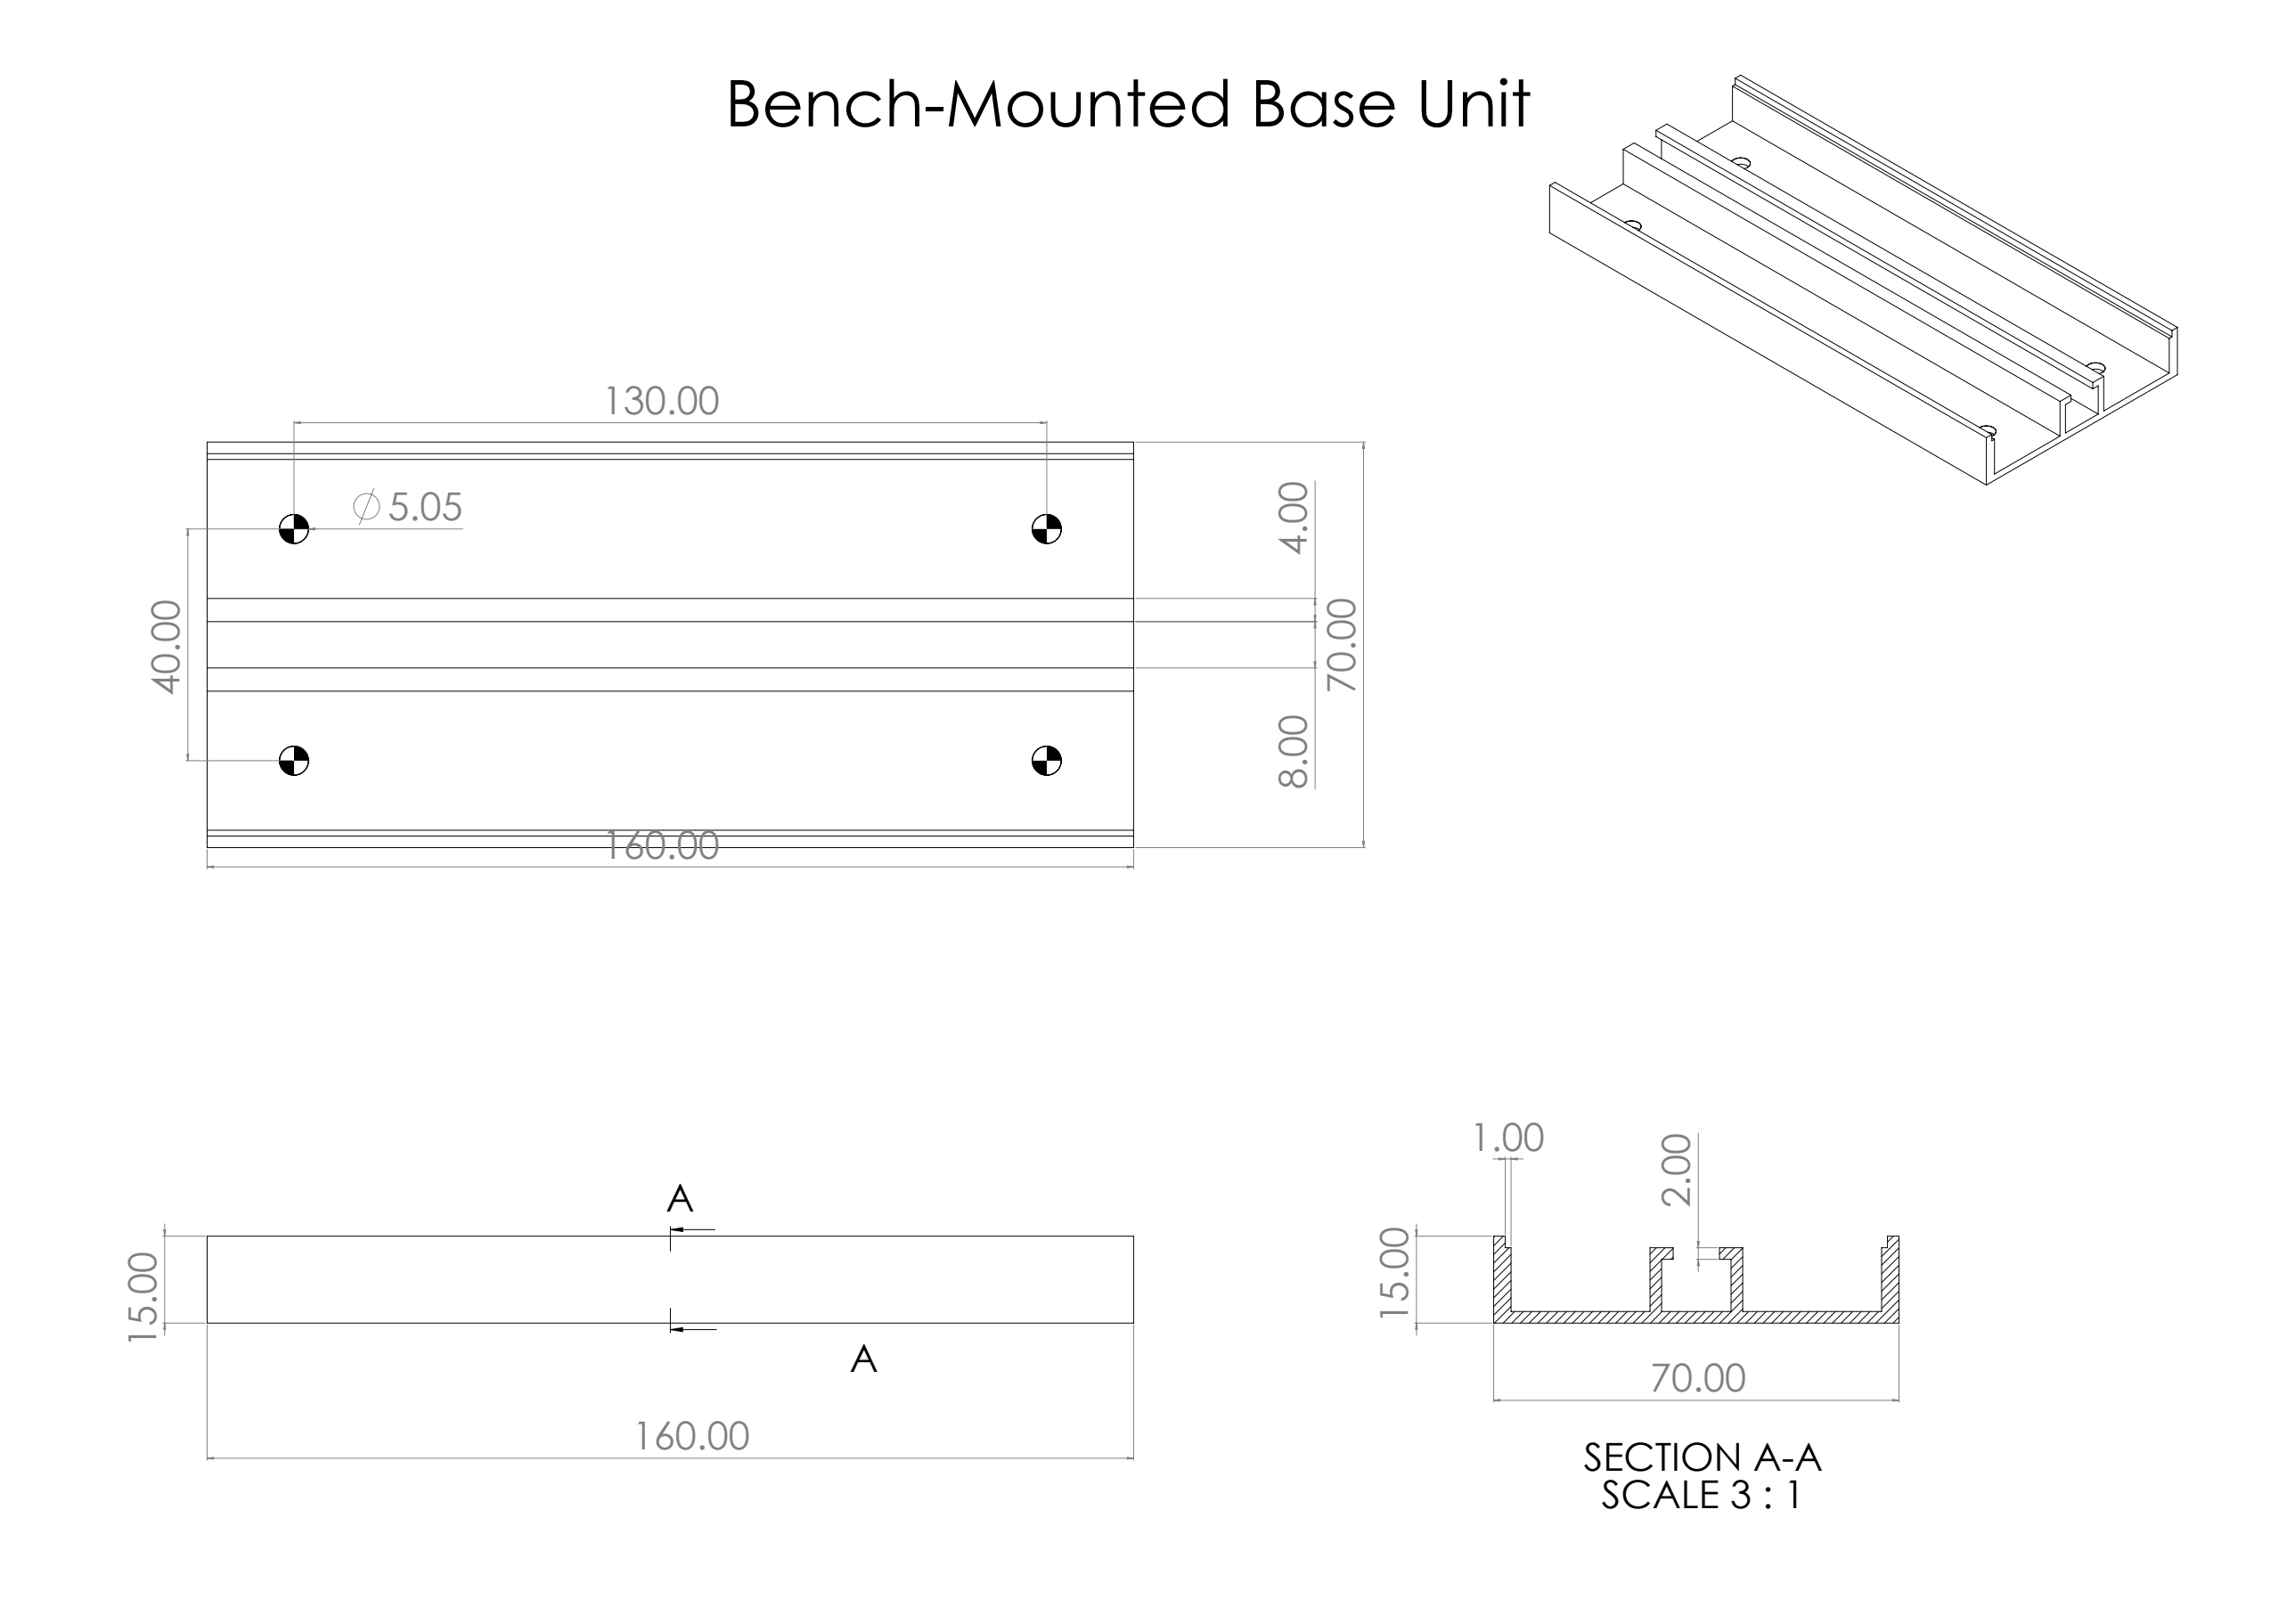
ISO-10303-21;
HEADER;
FILE_DESCRIPTION (('STEP AP214'),
    '1' );
FILE_NAME ('Bench-Mounted Base Unit.step',
    '2026-10-24T21:31:31',
    ( '' ),
    ( '' ),
    'SwSTEP 2.0',
    'SolidWorks 2025',
    '' );
FILE_SCHEMA (( 'AUTOMOTIVE_DESIGN' ));
ENDSEC;

DATA;
#19=ADVANCED_FACE ( 'NONE', ( #7663 ), #4110, .F. ) ;
#25=LINE ( 'NONE', #2406, #7510 ) ;
#36=DIRECTION ( 'NONE',  ( 0.000000000000000000, 0.000000000000000000, 1.000000000000000000 ) ) ;
#50=LINE ( 'NONE', #1350, #13702 ) ;
#81=VERTEX_POINT ( 'NONE', #9278 ) ;
#87=LINE ( 'NONE', #2465, #13317 ) ;
#98=ORIENTED_EDGE ( 'NONE', *, *, #8570, .T. ) ;
#157=EDGE_CURVE ( 'NONE', #531, #1580, #7972, .T. ) ;
#158=ADVANCED_FACE ( 'NONE', ( #10353 ), #436, .F. ) ;
#167=DIRECTION ( 'NONE',  ( -1.000000000000000000, 0.000000000000000000, 0.000000000000000000 ) ) ;
#177=AXIS2_PLACEMENT_3D ( 'NONE', #1271, #10901, #2354 ) ;
#186=EDGE_LOOP ( 'NONE', ( #1865, #4805, #14383, #1234 ) ) ;
#189=PRODUCT_DEFINITION_FORMATION_WITH_SPECIFIED_SOURCE ( 'ANY', '', #5935, .NOT_KNOWN. ) ;
#190=DIRECTION ( 'NONE',  ( -1.000000000000000000, -0.000000000000000000, -0.000000000000000000 ) ) ;
#205=ADVANCED_FACE ( 'NONE', ( #8045 ), #8050, .F. ) ;
#206=AXIS2_PLACEMENT_3D ( 'NONE', #6103, #12884, #8338 ) ;
#224=ORIENTED_EDGE ( 'NONE', *, *, #5040, .T. ) ;
#227=ORIENTED_EDGE ( 'NONE', *, *, #14224, .F. ) ;
#237=ORIENTED_EDGE ( 'NONE', *, *, #6908, .T. ) ;
#246=VERTEX_POINT ( 'NONE', #9730 ) ;
#280=LINE ( 'NONE', #11038, #4450 ) ;
#288=DIRECTION ( 'NONE',  ( 0.000000000000000000, -0.000000000000000000, -1.000000000000000000 ) ) ;
#292=EDGE_CURVE ( 'NONE', #5596, #3737, #9002, .T. ) ;
#295=ADVANCED_FACE ( 'NONE', ( #10164 ), #9788, .F. ) ;
#307=VERTEX_POINT ( 'NONE', #9085 ) ;
#313=CARTESIAN_POINT ( 'NONE',  ( 65.00000000000001421, -85.24929059928631148, 19.99999999999999645 ) ) ;
#341=VERTEX_POINT ( 'NONE', #685 ) ;
#395=EDGE_CURVE ( 'NONE', #2944, #14405, #10471, .T. ) ;
#404=VERTEX_POINT ( 'NONE', #7006 ) ;
#436=CONICAL_SURFACE ( 'NONE', #4856, 2.524999999999999467, 0.7853981633973787790 ) ;
#446=VERTEX_POINT ( 'NONE', #13931 ) ;
#450=EDGE_LOOP ( 'NONE', ( #14518, #14522, #9749, #6218 ) ) ;
#466=ADVANCED_FACE ( 'NONE', ( #3619 ), #3388, .F. ) ;
#475=VECTOR ( 'NONE', #11454, 1000.000000000000000 ) ;
#494=CARTESIAN_POINT ( 'NONE',  ( 80.00000000000001421, -72.24929059928631148, -32.99999999999999289 ) ) ;
#504=DIRECTION ( 'NONE',  ( -0.000000000000000000, 1.000000000000000000, 1.445602896647339163E-16 ) ) ;
#507=CARTESIAN_POINT ( 'NONE',  ( -80.00000000000001421, -74.24929059928631148, 8.000000000000001776 ) ) ;
#519=CARTESIAN_POINT ( 'NONE',  ( -80.00000000000001421, -72.24929059928631148, -32.99999999999999289 ) ) ;
#521=ORIENTED_EDGE ( 'NONE', *, *, #7499, .F. ) ;
#523=FACE_OUTER_BOUND ( 'NONE', #7005, .T. ) ;
#531=VERTEX_POINT ( 'NONE', #1686 ) ;
#538=VERTEX_POINT ( 'NONE', #9636 ) ;
#566=AXIS2_PLACEMENT_3D ( 'NONE', #4908, #5202, #14225 ) ;
#570=EDGE_CURVE ( 'NONE', #1671, #7867, #6379, .T. ) ;
#586=ORIENTED_EDGE ( 'NONE', *, *, #12573, .F. ) ;
#590=DIRECTION ( 'NONE',  ( 0.000000000000000000, 0.000000000000000000, 1.000000000000000000 ) ) ;
#592=DIRECTION ( 'NONE',  ( 0.000000000000000000, 0.7071067811865965336, 0.7071067811864985009 ) ) ;
#595=ADVANCED_FACE ( 'NONE', ( #523 ), #13090, .F. ) ;
#605=ORIENTED_EDGE ( 'NONE', *, *, #6309, .T. ) ;
#606=DIRECTION ( 'NONE',  ( -0.000000000000000000, 1.000000000000000000, 1.445602896647339163E-16 ) ) ;
#608=PLANE ( 'NONE',  #3506 ) ;
#634=DIRECTION ( 'NONE',  ( 0.000000000000000000, -0.000000000000000000, 1.000000000000000000 ) ) ;
#638=FACE_OUTER_BOUND ( 'NONE', #15061, .T. ) ;
#645=EDGE_CURVE ( 'NONE', #11420, #3697, #6168, .T. ) ;
#649=DIRECTION ( 'NONE',  ( 0.000000000000000000, 0.000000000000000000, -1.000000000000000000 ) ) ;
#671=CIRCLE ( 'NONE', #2885, 2.524999999999999467 ) ;
#685=CARTESIAN_POINT ( 'NONE',  ( -80.00000000000001421, -85.24929059928631148, 6.000000000000001776 ) ) ;
#699=ORIENTED_EDGE ( 'NONE', *, *, #13284, .T. ) ;
#712=DIRECTION ( 'NONE',  ( 8.659560562354330119E-17, 0.7071067811865966446, -0.7071067811864982788 ) ) ;
#715=EDGE_LOOP ( 'NONE', ( #1135, #7087, #13779, #14842 ) ) ;
#717=ORIENTED_EDGE ( 'NONE', *, *, #12868, .T. ) ;
#723=DIRECTION ( 'NONE',  ( 0.000000000000000000, 0.000000000000000000, 1.000000000000000000 ) ) ;
#725=AXIS2_PLACEMENT_3D ( 'NONE', #10060, #14667, #13517 ) ;
#726=ORIENTED_EDGE ( 'NONE', *, *, #9673, .T. ) ;
#732=CARTESIAN_POINT ( 'NONE',  ( 80.00000000000001421, -85.24929059928629727, -8.000000000000001776 ) ) ;
#733=DIRECTION ( 'NONE',  ( -1.000000000000000000, -0.000000000000000000, -0.000000000000000000 ) ) ;
#737=EDGE_CURVE ( 'NONE', #9321, #13009, #5442, .T. ) ;
#747=ORIENTED_EDGE ( 'NONE', *, *, #4471, .F. ) ;
#777=VERTEX_POINT ( 'NONE', #2331 ) ;
#784=VECTOR ( 'NONE', #14829, 1000.000000000000000 ) ;
#793=DIRECTION ( 'NONE',  ( -0.000000000000000000, 1.000000000000000000, 1.445602896647339163E-16 ) ) ;
#824=DIRECTION ( 'NONE',  ( 1.000000000000000000, 0.000000000000000000, 0.000000000000000000 ) ) ;
#831=ORIENTED_EDGE ( 'NONE', *, *, #11996, .T. ) ;
#839=DIRECTION ( 'NONE',  ( -0.000000000000000000, 0.000000000000000000, 1.000000000000000000 ) ) ;
#841=ADVANCED_FACE ( 'NONE', ( #12100 ), #14411, .F. ) ;
#866=VECTOR ( 'NONE', #2481, 1000.000000000000000 ) ;
#893=CARTESIAN_POINT ( 'NONE',  ( 65.00000000000001421, -87.24929059928631148, -19.99999999999999645 ) ) ;
#917=CARTESIAN_POINT ( 'NONE',  ( 65.00000000000001421, -85.24929059928629727, -19.99999999999999645 ) ) ;
#935=CARTESIAN_POINT ( 'NONE',  ( 80.00000000000001421, -74.24929059928631148, -4.000000000000000000 ) ) ;
#938=CARTESIAN_POINT ( 'NONE',  ( -65.00000000000001421, -85.24929059928629727, -19.99999999999999645 ) ) ;
#950=EDGE_CURVE ( 'NONE', #9272, #7803, #4209, .T. ) ;
#951=LINE ( 'NONE', #6885, #9647 ) ;
#960=CYLINDRICAL_SURFACE ( 'NONE', #11471, 2.499999999999995115 ) ;
#979=ORIENTED_EDGE ( 'NONE', *, *, #14140, .T. ) ;
#989=ADVANCED_FACE ( 'NONE', ( #7762 ), #6601, .F. ) ;
#995=DIRECTION ( 'NONE',  ( -1.000000000000000000, -0.000000000000000000, -0.000000000000000000 ) ) ;
#1008=FACE_OUTER_BOUND ( 'NONE', #715, .T. ) ;
#1018=LINE ( 'NONE', #2095, #4193 ) ;
#1029=DIRECTION ( 'NONE',  ( 0.000000000000000000, -1.000000000000000000, 1.927470528863120035E-16 ) ) ;
#1038=VECTOR ( 'NONE', #8723, 1000.000000000000000 ) ;
#1042=ORIENTED_EDGE ( 'NONE', *, *, #3581, .T. ) ;
#1046=VECTOR ( 'NONE', #9005, 1000.000000000000000 ) ;
#1058=DIRECTION ( 'NONE',  ( -0.000000000000000000, -1.000000000000000000, 4.625929269271485914E-16 ) ) ;
#1071=PLANE ( 'NONE',  #4829 ) ;
#1083=VERTEX_POINT ( 'NONE', #14148 ) ;
#1090=LINE ( 'NONE', #3173, #14166 ) ;
#1095=CARTESIAN_POINT ( 'NONE',  ( -80.00000000000001421, -74.24929059928631148, 32.99999999999999289 ) ) ;
#1135=ORIENTED_EDGE ( 'NONE', *, *, #12418, .T. ) ;
#1182=DIRECTION ( 'NONE',  ( 0.000000000000000000, 0.000000000000000000, 1.000000000000000000 ) ) ;
#1183=CIRCLE ( 'NONE', #7088, 2.499999999999995115 ) ;
#1184=VERTEX_POINT ( 'NONE', #1443 ) ;
#1186=EDGE_LOOP ( 'NONE', ( #7240, #3544 ) ) ;
#1209=LINE ( 'NONE', #4592, #1781 ) ;
#1234=ORIENTED_EDGE ( 'NONE', *, *, #15073, .T. ) ;
#1237=EDGE_CURVE ( 'NONE', #11933, #12860, #5235, .T. ) ;
#1245=ORIENTED_EDGE ( 'NONE', *, *, #645, .F. ) ;
#1246=DIRECTION ( 'NONE',  ( 0.000000000000000000, 0.000000000000000000, 1.000000000000000000 ) ) ;
#1271=CARTESIAN_POINT ( 'NONE',  ( 80.00000000000001421, -85.24929059928629727, 32.00000000000000000 ) ) ;
#1274=ORIENTED_EDGE ( 'NONE', *, *, #4240, .F. ) ;
#1285=VECTOR ( 'NONE', #3850, 1000.000000000000000 ) ;
#1296=EDGE_CURVE ( 'NONE', #3181, #6626, #5246, .T. ) ;
#1311=VERTEX_POINT ( 'NONE', #9697 ) ;
#1316=FACE_OUTER_BOUND ( 'NONE', #2115, .T. ) ;
#1323=ORIENTED_EDGE ( 'NONE', *, *, #13700, .F. ) ;
#1329=ADVANCED_FACE ( 'NONE', ( #5059 ), #3895, .F. ) ;
#1330=DIRECTION ( 'NONE',  ( -1.000000000000000000, -0.000000000000000000, -0.000000000000000000 ) ) ;
#1350=CARTESIAN_POINT ( 'NONE',  ( 80.00000000000001421, -85.24929059928629727, 8.000000000000001776 ) ) ;
#1389=ORIENTED_EDGE ( 'NONE', *, *, #12424, .F. ) ;
#1407=ADVANCED_FACE ( 'NONE', ( #7894 ), #8810, .F. ) ;
#1413=CARTESIAN_POINT ( 'NONE',  ( 80.00000000000001421, -76.24929059928631148, -6.000000000000000000 ) ) ;
#1417=FACE_OUTER_BOUND ( 'NONE', #2786, .T. ) ;
#1430=EDGE_CURVE ( 'NONE', #4665, #307, #15084, .T. ) ;
#1443=CARTESIAN_POINT ( 'NONE',  ( -80.00000000000001421, -76.24929059928631148, -6.000000000000000000 ) ) ;
#1452=AXIS2_PLACEMENT_3D ( 'NONE', #11065, #9559, #2549 ) ;
#1456=ORIENTED_EDGE ( 'NONE', *, *, #10701, .T. ) ;
#1465=DIRECTION ( 'NONE',  ( 0.000000000000000000, -1.000000000000000000, 0.000000000000000000 ) ) ;
#1466=DIRECTION ( 'NONE',  ( -1.000000000000000000, -0.000000000000000000, -0.000000000000000000 ) ) ;
#1471=VECTOR ( 'NONE', #995, 1000.000000000000000 ) ;
#1479=EDGE_CURVE ( 'NONE', #5596, #6896, #5906, .T. ) ;
#1480=DIRECTION ( 'NONE',  ( -0.000000000000000000, 1.000000000000000000, 1.445602896647339163E-16 ) ) ;
#1490=DIRECTION ( 'NONE',  ( -0.000000000000000000, 1.000000000000000000, -0.000000000000000000 ) ) ;
#1491=CARTESIAN_POINT ( 'NONE',  ( 65.00000000000001421, -85.24929059928629727, -22.52499999999999503 ) ) ;
#1552=CARTESIAN_POINT ( 'NONE',  ( 80.00000000000001421, -76.24929059928631148, -4.000000000000000000 ) ) ;
#1571=( NAMED_UNIT ( * ) PLANE_ANGLE_UNIT ( ) SI_UNIT ( $, .RADIAN. ) );
#1580=VERTEX_POINT ( 'NONE', #13813 ) ;
#1584=DIRECTION ( 'NONE',  ( -1.000000000000000000, -0.000000000000000000, -0.000000000000000000 ) ) ;
#1589=PLANE ( 'NONE',  #10650 ) ;
#1604=EDGE_CURVE ( 'NONE', #12366, #3697, #9209, .T. ) ;
#1615=ORIENTED_EDGE ( 'NONE', *, *, #2520, .F. ) ;
#1636=( NAMED_UNIT ( * ) SI_UNIT ( $, .STERADIAN. ) SOLID_ANGLE_UNIT ( ) );
#1638=SHAPE_REPRESENTATION_RELATIONSHIP ( 'NONE' , 'NONE' ,  #11466, #10707 ) ;
#1644=AXIS2_PLACEMENT_3D ( 'NONE', #14275, #15068, #3574 ) ;
#1645=AXIS2_PLACEMENT_3D ( 'NONE', #14043, #15199, #1029 ) ;
#1668=VECTOR ( 'NONE', #10391, 1000.000000000000000 ) ;
#1671=VERTEX_POINT ( 'NONE', #11398 ) ;
#1683=ORIENTED_EDGE ( 'NONE', *, *, #7122, .F. ) ;
#1686=CARTESIAN_POINT ( 'NONE',  ( -80.00000000000001421, -74.24929059928631148, -8.000000000000001776 ) ) ;
#1689=EDGE_LOOP ( 'NONE', ( #1895, #13919 ) ) ;
#1696=DIRECTION ( 'NONE',  ( 0.000000000000000000, 1.000000000000000000, 0.000000000000000000 ) ) ;
#1706=VECTOR ( 'NONE', #9108, 1000.000000000000000 ) ;
#1722=ORIENTED_EDGE ( 'NONE', *, *, #13799, .T. ) ;
#1724=CARTESIAN_POINT ( 'NONE',  ( 80.00000000000001421, -85.24929059928631148, -6.000000000000001776 ) ) ;
#1745=AXIS2_PLACEMENT_3D ( 'NONE', #3312, #839, #5548 ) ;
#1750=CARTESIAN_POINT ( 'NONE',  ( 65.00000000000001421, -87.24929059928631148, -17.50000000000000000 ) ) ;
#1752=ORIENTED_EDGE ( 'NONE', *, *, #14178, .F. ) ;
#1758=ORIENTED_EDGE ( 'NONE', *, *, #7122, .T. ) ;
#1766=VECTOR ( 'NONE', #7495, 1000.000000000000000 ) ;
#1781=VECTOR ( 'NONE', #5838, 1000.000000000000000 ) ;
#1800=VECTOR ( 'NONE', #3512, 1000.000000000000000 ) ;
#1814=CARTESIAN_POINT ( 'NONE',  ( 80.00000000000001421, -74.24929059928631148, 32.00000000000000000 ) ) ;
#1825=DIRECTION ( 'NONE',  ( -1.000000000000000000, -0.000000000000000000, -0.000000000000000000 ) ) ;
#1827=LINE ( 'NONE', #519, #6922 ) ;
#1843=EDGE_CURVE ( 'NONE', #3737, #2170, #10798, .T. ) ;
#1859=DIRECTION ( 'NONE',  ( -1.000000000000000000, -0.000000000000000000, -0.000000000000000000 ) ) ;
#1863=VERTEX_POINT ( 'NONE', #9494 ) ;
#1865=ORIENTED_EDGE ( 'NONE', *, *, #645, .T. ) ;
#1878=VECTOR ( 'NONE', #4733, 1000.000000000000000 ) ;
#1880=FACE_OUTER_BOUND ( 'NONE', #12072, .T. ) ;
#1888=EDGE_LOOP ( 'NONE', ( #8253, #2831, #13213, #11548 ) ) ;
#1895=ORIENTED_EDGE ( 'NONE', *, *, #14224, .T. ) ;
#1917=CARTESIAN_POINT ( 'NONE',  ( 80.00000000000001421, -85.24929059928629727, -32.00000000000000000 ) ) ;
#1918=VERTEX_POINT ( 'NONE', #4502 ) ;
#1919=DIRECTION ( 'NONE',  ( 0.000000000000000000, 0.000000000000000000, 1.000000000000000000 ) ) ;
#1937=VECTOR ( 'NONE', #1859, 1000.000000000000000 ) ;
#1966=CARTESIAN_POINT ( 'NONE',  ( 80.00000000000001421, -74.24929059928631148, 4.000000000000000000 ) ) ;
#1978=VERTEX_POINT ( 'NONE', #9357 ) ;
#1999=VECTOR ( 'NONE', #1490, 1000.000000000000000 ) ;
#2012=AXIS2_PLACEMENT_3D ( 'NONE', #10249, #6482, #7789 ) ;
#2026=VECTOR ( 'NONE', #8584, 1000.000000000000000 ) ;
#2032=LINE ( 'NONE', #10277, #9994 ) ;
#2049=CARTESIAN_POINT ( 'NONE',  ( -65.00000000000001421, -85.24929059928631148, 19.99999999999999645 ) ) ;
#2050=ORIENTED_EDGE ( 'NONE', *, *, #12034, .T. ) ;
#2054=DIRECTION ( 'NONE',  ( -1.000000000000000000, -0.000000000000000000, -0.000000000000000000 ) ) ;
#2060=DIRECTION ( 'NONE',  ( 8.659560562354330119E-17, 0.7071067811865966446, -0.7071067811864982788 ) ) ;
#2095=CARTESIAN_POINT ( 'NONE',  ( 80.00000000000001421, -74.24929059928631148, -8.000000000000001776 ) ) ;
#2110=CARTESIAN_POINT ( 'NONE',  ( -65.00000000000001421, -85.24929059928631148, 19.99999999999999645 ) ) ;
#2115=EDGE_LOOP ( 'NONE', ( #2607, #14282, #14380, #13821 ) ) ;
#2126=CARTESIAN_POINT ( 'NONE',  ( -80.00000000000001421, -74.24929059928631148, -32.99999999999999289 ) ) ;
#2127=CARTESIAN_POINT ( 'NONE',  ( 80.00000000000001421, -74.24929059928631148, 32.99999999999999289 ) ) ;
#2142=CARTESIAN_POINT ( 'NONE',  ( 65.00000000000001421, -87.24929059928631148, -19.99999999999999645 ) ) ;
#2151=DIRECTION ( 'NONE',  ( 0.000000000000000000, 1.000000000000000000, 1.927470528863120035E-16 ) ) ;
#2153=CARTESIAN_POINT ( 'NONE',  ( 80.00000000000001421, -85.24929059928629727, 32.00000000000000000 ) ) ;
#2158=ORIENTED_EDGE ( 'NONE', *, *, #4168, .T. ) ;
#2164=DIRECTION ( 'NONE',  ( -0.000000000000000000, 1.000000000000000000, 1.445602896647339163E-16 ) ) ;
#2170=VERTEX_POINT ( 'NONE', #14207 ) ;
#2186=CARTESIAN_POINT ( 'NONE',  ( 65.00000000000001421, -85.27429059928630295, 22.50000000000000000 ) ) ;
#2202=CARTESIAN_POINT ( 'NONE',  ( -80.00000000000001421, -72.24929059928631148, 34.99999999999999289 ) ) ;
#2222=DIRECTION ( 'NONE',  ( 0.000000000000000000, 1.000000000000000000, 0.000000000000000000 ) ) ;
#2246=DIRECTION ( 'NONE',  ( 0.000000000000000000, -1.000000000000000000, -4.625929269271485914E-16 ) ) ;
#2249=DIRECTION ( 'NONE',  ( 0.000000000000000000, 0.000000000000000000, 1.000000000000000000 ) ) ;
#2268=CIRCLE ( 'NONE', #10878, 2.524999999999999467 ) ;
#2279=ADVANCED_FACE ( 'NONE', ( #7007 ), #14950, .F. ) ;
#2290=CARTESIAN_POINT ( 'NONE',  ( -65.00000000000001421, -85.24929059928629727, -19.99999999999999645 ) ) ;
#2293=VECTOR ( 'NONE', #12378, 1000.000000000000114 ) ;
#2310=ADVANCED_FACE ( 'NONE', ( #5628 ), #10397, .F. ) ;
#2322=DIRECTION ( 'NONE',  ( 0.000000000000000000, 0.000000000000000000, 1.000000000000000000 ) ) ;
#2330=CARTESIAN_POINT ( 'NONE',  ( 65.00000000000001421, -85.24929059928631148, 17.50000000000000000 ) ) ;
#2331=CARTESIAN_POINT ( 'NONE',  ( -65.00000000000001421, -85.24929059928631148, 22.52499999999999503 ) ) ;
#2344=LINE ( 'NONE', #3502, #12602 ) ;
#2354=DIRECTION ( 'NONE',  ( 0.000000000000000000, -1.445602896647339410E-16, -1.000000000000000000 ) ) ;
#2355=ADVANCED_FACE ( 'NONE', ( #12549 ), #6693, .F. ) ;
#2357=EDGE_CURVE ( 'NONE', #2753, #3972, #8006, .T. ) ;
#2380=CARTESIAN_POINT ( 'NONE',  ( 80.00000000000001421, -76.24929059928631148, 4.000000000000000000 ) ) ;
#2382=EDGE_LOOP ( 'NONE', ( #1456, #9704, #14086, #14524 ) ) ;
#2406=CARTESIAN_POINT ( 'NONE',  ( 80.00000000000001421, -76.24929059928631148, -6.000000000000000000 ) ) ;
#2419=DIRECTION ( 'NONE',  ( -0.000000000000000000, 1.000000000000000000, 1.445602896647339163E-16 ) ) ;
#2465=CARTESIAN_POINT ( 'NONE',  ( -80.00000000000001421, -85.24929059928629727, -32.00000000000000000 ) ) ;
#2471=CARTESIAN_POINT ( 'NONE',  ( 80.00000000000001421, -76.24929059928631148, 4.000000000000000000 ) ) ;
#2481=DIRECTION ( 'NONE',  ( -0.000000000000000000, -0.000000000000000000, 1.000000000000000000 ) ) ;
#2487=AXIS2_PLACEMENT_3D ( 'NONE', #5138, #3973, #3903 ) ;
#2491=ORIENTED_EDGE ( 'NONE', *, *, #11907, .T. ) ;
#2520=EDGE_CURVE ( 'NONE', #10741, #11420, #9637, .T. ) ;
#2525=VECTOR ( 'NONE', #2575, 1000.000000000000000 ) ;
#2547=EDGE_LOOP ( 'NONE', ( #6515, #3993 ) ) ;
#2549=DIRECTION ( 'NONE',  ( 0.000000000000000000, 1.000000000000000000, -4.625929269271485914E-16 ) ) ;
#2567=FACE_OUTER_BOUND ( 'NONE', #7297, .T. ) ;
#2575=DIRECTION ( 'NONE',  ( 0.000000000000000000, 0.000000000000000000, -1.000000000000000000 ) ) ;
#2577=CARTESIAN_POINT ( 'NONE',  ( -65.00000000000001421, -85.24929059928631148, 17.50000000000000000 ) ) ;
#2586=UNCERTAINTY_MEASURE_WITH_UNIT (LENGTH_MEASURE( 1.000000000000000082E-05 ), #3939, 'distance_accuracy_value', 'NONE');
#2589=VERTEX_POINT ( 'NONE', #12224 ) ;
#2601=EDGE_CURVE ( 'NONE', #14307, #7867, #11002, .T. ) ;
#2607=ORIENTED_EDGE ( 'NONE', *, *, #6790, .F. ) ;
#2670=EDGE_LOOP ( 'NONE', ( #15221, #586, #6959, #4327 ) ) ;
#2675=ORIENTED_EDGE ( 'NONE', *, *, #5963, .T. ) ;
#2677=CARTESIAN_POINT ( 'NONE',  ( -65.00000000000001421, -85.24929059928631148, 17.47499999999999787 ) ) ;
#2679=PLANE ( 'NONE',  #2487 ) ;
#2698=ORIENTED_EDGE ( 'NONE', *, *, #14591, .F. ) ;
#2700=LINE ( 'NONE', #1552, #4226 ) ;
#2720=DIRECTION ( 'NONE',  ( 0.000000000000000000, -0.000000000000000000, -1.000000000000000000 ) ) ;
#2729=UNCERTAINTY_MEASURE_WITH_UNIT (LENGTH_MEASURE( 1.000000000000000082E-05 ), #6118, 'distance_accuracy_value', 'NONE');
#2731=DIRECTION ( 'NONE',  ( -0.000000000000000000, 1.000000000000000000, 1.445602896647339163E-16 ) ) ;
#2751=ORIENTED_EDGE ( 'NONE', *, *, #10179, .F. ) ;
#2753=VERTEX_POINT ( 'NONE', #5431 ) ;
#2781=CARTESIAN_POINT ( 'NONE',  ( -80.00000000000001421, -87.24929059928629727, 0.000000000000000000 ) ) ;
#2786=EDGE_LOOP ( 'NONE', ( #13073, #9483, #7592, #3260 ) ) ;
#2804=CARTESIAN_POINT ( 'NONE',  ( 80.00000000000001421, -76.24929059928631148, 6.000000000000000000 ) ) ;
#2831=ORIENTED_EDGE ( 'NONE', *, *, #1296, .F. ) ;
#2845=FACE_OUTER_BOUND ( 'NONE', #7939, .T. ) ;
#2885=AXIS2_PLACEMENT_3D ( 'NONE', #3967, #504, #14517 ) ;
#2892=DIRECTION ( 'NONE',  ( 1.000000000000000000, 0.000000000000000000, 0.000000000000000000 ) ) ;
#2923=EDGE_CURVE ( 'NONE', #3601, #1918, #7158, .T. ) ;
#2938=ORIENTED_EDGE ( 'NONE', *, *, #12012, .T. ) ;
#2941=VECTOR ( 'NONE', #5173, 1000.000000000000000 ) ;
#2944=VERTEX_POINT ( 'NONE', #13276 ) ;
#2954=LINE ( 'NONE', #8714, #5680 ) ;
#2965=CARTESIAN_POINT ( 'NONE',  ( 80.00000000000001421, -72.24929059928631148, -34.99999999999999289 ) ) ;
#3011=VERTEX_POINT ( 'NONE', #8791 ) ;
#3018=ORIENTED_EDGE ( 'NONE', *, *, #2923, .F. ) ;
#3022=EDGE_CURVE ( 'NONE', #7867, #1978, #2954, .T. ) ;
#3037=AXIS2_PLACEMENT_3D ( 'NONE', #4264, #11343, #6733 ) ;
#3042=CARTESIAN_POINT ( 'NONE',  ( 80.00000000000001421, -85.24929059928629727, 8.000000000000001776 ) ) ;
#3051=DIRECTION ( 'NONE',  ( 0.000000000000000000, 0.000000000000000000, 1.000000000000000000 ) ) ;
#3066=DIRECTION ( 'NONE',  ( -1.000000000000000000, -0.000000000000000000, -0.000000000000000000 ) ) ;
#3068=EDGE_CURVE ( 'NONE', #3756, #446, #14953, .T. ) ;
#3075=ORIENTED_EDGE ( 'NONE', *, *, #13143, .F. ) ;
#3095=CARTESIAN_POINT ( 'NONE',  ( 80.00000000000001421, -76.24929059928631148, 6.000000000000000000 ) ) ;
#3106=EDGE_CURVE ( 'NONE', #1863, #1580, #7956, .T. ) ;
#3110=VERTEX_POINT ( 'NONE', #3095 ) ;
#3121=ORIENTED_EDGE ( 'NONE', *, *, #3711, .F. ) ;
#3133=VECTOR ( 'NONE', #5474, 1000.000000000000000 ) ;
#3135=CARTESIAN_POINT ( 'NONE',  ( -65.00000000000001421, -85.27429059928630295, 19.99999999999999645 ) ) ;
#3161=CARTESIAN_POINT ( 'NONE',  ( 80.00000000000001421, -72.24929059928631148, 34.99999999999999289 ) ) ;
#3173=CARTESIAN_POINT ( 'NONE',  ( 80.00000000000001421, -74.24929059928631148, 32.00000000000000000 ) ) ;
#3181=VERTEX_POINT ( 'NONE', #11714 ) ;
#3204=CARTESIAN_POINT ( 'NONE',  ( -65.00000000000001421, -85.27429059928630295, 22.50000000000000000 ) ) ;
#3240=ADVANCED_FACE ( 'NONE', ( #2567 ), #10799, .F. ) ;
#3260=ORIENTED_EDGE ( 'NONE', *, *, #14534, .T. ) ;
#3262=VERTEX_POINT ( 'NONE', #12808 ) ;
#3300=DIRECTION ( 'NONE',  ( 0.000000000000000000, 0.000000000000000000, 1.000000000000000000 ) ) ;
#3306=ORIENTED_EDGE ( 'NONE', *, *, #12717, .F. ) ;
#3312=CARTESIAN_POINT ( 'NONE',  ( 80.00000000000001421, -74.24929059928631148, 4.000000000000000000 ) ) ;
#3322=CARTESIAN_POINT ( 'NONE',  ( -80.00000000000001421, -72.24929059928631148, -32.99999999999999289 ) ) ;
#3334=AXIS2_PLACEMENT_3D ( 'NONE', #7174, #8340, #1246 ) ;
#3366=( GEOMETRIC_REPRESENTATION_CONTEXT ( 3 ) GLOBAL_UNCERTAINTY_ASSIGNED_CONTEXT ( ( #2586 ) ) GLOBAL_UNIT_ASSIGNED_CONTEXT ( ( #3939, #1571, #4958 ) ) REPRESENTATION_CONTEXT ( 'NONE', 'WORKASPACE' ) );
#3369=CARTESIAN_POINT ( 'NONE',  ( 80.00000000000001421, -87.24929059928631148, 35.00000000000000000 ) ) ;
#3372=FACE_OUTER_BOUND ( 'NONE', #2382, .T. ) ;
#3385=EDGE_CURVE ( 'NONE', #12875, #1311, #15226, .T. ) ;
#3388=PLANE ( 'NONE',  #14203 ) ;
#3411=DIRECTION ( 'NONE',  ( -1.000000000000000000, 0.000000000000000000, -0.000000000000000000 ) ) ;
#3425=AXIS2_PLACEMENT_3D ( 'NONE', #7024, #3563, #3411 ) ;
#3435=EDGE_CURVE ( 'NONE', #538, #5126, #9087, .T. ) ;
#3502=CARTESIAN_POINT ( 'NONE',  ( 80.00000000000001421, -74.24929059928631148, -32.00000000000000000 ) ) ;
#3506=AXIS2_PLACEMENT_3D ( 'NONE', #8845, #10008, #11079 ) ;
#3512=DIRECTION ( 'NONE',  ( -1.000000000000000000, -0.000000000000000000, -0.000000000000000000 ) ) ;
#3514=DIRECTION ( 'NONE',  ( -0.000000000000000000, -1.000000000000000000, -0.000000000000000000 ) ) ;
#3540=FACE_OUTER_BOUND ( 'NONE', #7300, .T. ) ;
#3544=ORIENTED_EDGE ( 'NONE', *, *, #7499, .T. ) ;
#3563=DIRECTION ( 'NONE',  ( 0.000000000000000000, 0.000000000000000000, -1.000000000000000000 ) ) ;
#3574=DIRECTION ( 'NONE',  ( 0.000000000000000000, -0.000000000000000000, 1.000000000000000000 ) ) ;
#3581=EDGE_CURVE ( 'NONE', #446, #7966, #5251, .T. ) ;
#3589=ORIENTED_EDGE ( 'NONE', *, *, #14866, .F. ) ;
#3599=VECTOR ( 'NONE', #14599, 1000.000000000000000 ) ;
#3600=ORIENTED_EDGE ( 'NONE', *, *, #6884, .T. ) ;
#3601=VERTEX_POINT ( 'NONE', #15015 ) ;
#3602=CONICAL_SURFACE ( 'NONE', #7532, 2.524999999999999467, 0.7853981633973787790 ) ;
#3619=FACE_OUTER_BOUND ( 'NONE', #11346, .T. ) ;
#3622=LINE ( 'NONE', #13311, #11142 ) ;
#3636=CYLINDRICAL_SURFACE ( 'NONE', #206, 2.499999999999995115 ) ;
#3639=LINE ( 'NONE', #2330, #8988 ) ;
#3656=AXIS2_PLACEMENT_3D ( 'NONE', #8168, #9399, #4459 ) ;
#3659=DIRECTION ( 'NONE',  ( 0.000000000000000000, 0.7071067811865965336, 0.7071067811864985009 ) ) ;
#3675=CARTESIAN_POINT ( 'NONE',  ( 65.00000000000001421, -87.24929059928631148, 19.99999999999999645 ) ) ;
#3676=AXIS2_PLACEMENT_3D ( 'NONE', #8702, #5248, #14621 ) ;
#3681=ORIENTED_EDGE ( 'NONE', *, *, #12056, .T. ) ;
#3683=ORIENTED_EDGE ( 'NONE', *, *, #14758, .T. ) ;
#3692=DIRECTION ( 'NONE',  ( -1.000000000000000000, -0.000000000000000000, -0.000000000000000000 ) ) ;
#3697=VERTEX_POINT ( 'NONE', #12766 ) ;
#3699=VECTOR ( 'NONE', #15100, 1000.000000000000000 ) ;
#3711=EDGE_CURVE ( 'NONE', #446, #5596, #11513, .T. ) ;
#3718=DIRECTION ( 'NONE',  ( 0.000000000000000000, -1.000000000000000000, 0.000000000000000000 ) ) ;
#3730=EDGE_CURVE ( 'NONE', #15028, #1311, #13679, .T. ) ;
#3734=AXIS2_PLACEMENT_3D ( 'NONE', #2142, #2222, #3300 ) ;
#3737=VERTEX_POINT ( 'NONE', #12682 ) ;
#3756=VERTEX_POINT ( 'NONE', #12446 ) ;
#3771=DIRECTION ( 'NONE',  ( 0.000000000000000000, 0.000000000000000000, 1.000000000000000000 ) ) ;
#3775=AXIS2_PLACEMENT_3D ( 'NONE', #7091, #5010, #3771 ) ;
#3784=FACE_OUTER_BOUND ( 'NONE', #9288, .T. ) ;
#3794=FACE_OUTER_BOUND ( 'NONE', #2670, .T. ) ;
#3809=ORIENTED_EDGE ( 'NONE', *, *, #1479, .T. ) ;
#3822=ORIENTED_EDGE ( 'NONE', *, *, #12731, .F. ) ;
#3833=EDGE_LOOP ( 'NONE', ( #12228, #6363, #10709, #13289 ) ) ;
#3835=DIRECTION ( 'NONE',  ( 0.000000000000000000, 0.000000000000000000, 1.000000000000000000 ) ) ;
#3837=CARTESIAN_POINT ( 'NONE',  ( -80.00000000000001421, -74.24929059928631148, 8.000000000000001776 ) ) ;
#3846=ORIENTED_EDGE ( 'NONE', *, *, #950, .T. ) ;
#3850=DIRECTION ( 'NONE',  ( 0.000000000000000000, 1.000000000000000000, 4.625929269271485914E-16 ) ) ;
#3852=DIRECTION ( 'NONE',  ( 0.000000000000000000, -1.000000000000000000, 0.000000000000000000 ) ) ;
#3858=VECTOR ( 'NONE', #8478, 1000.000000000000000 ) ;
#3895=PLANE ( 'NONE',  #13847 ) ;
#3903=DIRECTION ( 'NONE',  ( -1.000000000000000000, 0.000000000000000000, -0.000000000000000000 ) ) ;
#3938=CARTESIAN_POINT ( 'NONE',  ( 80.00000000000001421, -72.24929059928631148, -32.99999999999999289 ) ) ;
#3939=( LENGTH_UNIT ( ) NAMED_UNIT ( * ) SI_UNIT ( .MILLI., .METRE. ) );
#3956=ORIENTED_EDGE ( 'NONE', *, *, #13284, .F. ) ;
#3959=ORIENTED_EDGE ( 'NONE', *, *, #13050, .T. ) ;
#3961=AXIS2_PLACEMENT_3D ( 'NONE', #10487, #12804, #2249 ) ;
#3967=CARTESIAN_POINT ( 'NONE',  ( 65.00000000000001421, -85.24929059928631148, 19.99999999999999645 ) ) ;
#3972=VERTEX_POINT ( 'NONE', #1095 ) ;
#3973=DIRECTION ( 'NONE',  ( 0.000000000000000000, 0.000000000000000000, -1.000000000000000000 ) ) ;
#3992=DIRECTION ( 'NONE',  ( 0.000000000000000000, 1.000000000000000000, 0.000000000000000000 ) ) ;
#3993=ORIENTED_EDGE ( 'NONE', *, *, #2923, .T. ) ;
#3996=CARTESIAN_POINT ( 'NONE',  ( 80.00000000000001421, -76.24929059928631148, -6.000000000000000000 ) ) ;
#4031=EDGE_CURVE ( 'NONE', #246, #1863, #1018, .T. ) ;
#4033=ADVANCED_FACE ( 'NONE', ( #6789 ), #11479, .F. ) ;
#4038=VERTEX_POINT ( 'NONE', #15035 ) ;
#4082=CARTESIAN_POINT ( 'NONE',  ( 0.000000000000000000, 0.000000000000000000, 0.000000000000000000 ) ) ;
#4096=VERTEX_POINT ( 'NONE', #7119 ) ;
#4110=CYLINDRICAL_SURFACE ( 'NONE', #8317, 2.499999999999995115 ) ;
#4137=EDGE_LOOP ( 'NONE', ( #3075, #12175, #3600, #10609 ) ) ;
#4159=CONICAL_SURFACE ( 'NONE', #13037, 2.524999999999999467, 0.7853981633973787790 ) ;
#4164=ORIENTED_EDGE ( 'NONE', *, *, #6398, .T. ) ;
#4168=EDGE_CURVE ( 'NONE', #3262, #341, #951, .T. ) ;
#4193=VECTOR ( 'NONE', #1182, 1000.000000000000000 ) ;
#4209=LINE ( 'NONE', #4367, #2293 ) ;
#4212=CARTESIAN_POINT ( 'NONE',  ( -65.00000000000001421, -87.24929059928631148, -19.99999999999999645 ) ) ;
#4214=ORIENTED_EDGE ( 'NONE', *, *, #4031, .F. ) ;
#4218=ADVANCED_FACE ( 'NONE', ( #12903 ), #12030, .F. ) ;
#4221=DIRECTION ( 'NONE',  ( 0.000000000000000000, 0.000000000000000000, 1.000000000000000000 ) ) ;
#4226=VECTOR ( 'NONE', #6256, 1000.000000000000000 ) ;
#4236=LINE ( 'NONE', #4394, #3699 ) ;
#4240=EDGE_CURVE ( 'NONE', #3262, #3110, #9743, .T. ) ;
#4243=ORIENTED_EDGE ( 'NONE', *, *, #4577, .F. ) ;
#4245=DIRECTION ( 'NONE',  ( -0.000000000000000000, 1.734723475976817547E-15, 1.000000000000000000 ) ) ;
#4264=CARTESIAN_POINT ( 'NONE',  ( 65.00000000000001421, -85.27429059928628874, -19.99999999999999645 ) ) ;
#4313=CARTESIAN_POINT ( 'NONE',  ( 65.00000000000001421, -85.27429059928628874, -17.49999999999999645 ) ) ;
#4325=EDGE_LOOP ( 'NONE', ( #13818, #7388, #6167, #10076 ) ) ;
#4327=ORIENTED_EDGE ( 'NONE', *, *, #13432, .T. ) ;
#4328=DIRECTION ( 'NONE',  ( 0.000000000000000000, 1.000000000000000000, 0.000000000000000000 ) ) ;
#4332=PLANE ( 'NONE',  #1645 ) ;
#4334=VECTOR ( 'NONE', #11031, 1000.000000000000000 ) ;
#4355=AXIS2_PLACEMENT_3D ( 'NONE', #12361, #649, #7590 ) ;
#4367=CARTESIAN_POINT ( 'NONE',  ( -65.00000000000001421, -85.24929059928631148, 17.47499999999999787 ) ) ;
#4379=CARTESIAN_POINT ( 'NONE',  ( 80.00000000000001421, -74.24929059928631148, -32.99999999999999289 ) ) ;
#4380=CARTESIAN_POINT ( 'NONE',  ( -80.00000000000001421, -85.24929059928629727, 32.00000000000000000 ) ) ;
#4394=CARTESIAN_POINT ( 'NONE',  ( 80.00000000000001421, -74.24929059928631148, 32.00000000000000000 ) ) ;
#4402=CARTESIAN_POINT ( 'NONE',  ( 80.00000000000001421, -72.24929059928631148, 34.99999999999999289 ) ) ;
#4413=DIRECTION ( 'NONE',  ( 0.000000000000000000, 0.000000000000000000, 1.000000000000000000 ) ) ;
#4450=VECTOR ( 'NONE', #2731, 1000.000000000000000 ) ;
#4459=DIRECTION ( 'NONE',  ( 0.000000000000000000, 0.000000000000000000, 1.000000000000000000 ) ) ;
#4471=EDGE_CURVE ( 'NONE', #8897, #777, #10699, .T. ) ;
#4479=AXIS2_PLACEMENT_3D ( 'NONE', #10431, #10347, #4413 ) ;
#4482=AXIS2_PLACEMENT_3D ( 'NONE', #14023, #8414, #14183 ) ;
#4487=DIRECTION ( 'NONE',  ( -0.000000000000000000, 1.000000000000000000, 1.445602896647339163E-16 ) ) ;
#4491=VECTOR ( 'NONE', #11885, 1000.000000000000000 ) ;
#4502=CARTESIAN_POINT ( 'NONE',  ( -65.00000000000001421, -87.24929059928631148, 22.49999999999999289 ) ) ;
#4507=CIRCLE ( 'NONE', #13124, 2.524999999999999467 ) ;
#4510=ORIENTED_EDGE ( 'NONE', *, *, #12868, .F. ) ;
#4556=EDGE_CURVE ( 'NONE', #7720, #14080, #7232, .T. ) ;
#4577=EDGE_CURVE ( 'NONE', #341, #2589, #10468, .T. ) ;
#4592=CARTESIAN_POINT ( 'NONE',  ( 80.00000000000001421, -74.24929059928631148, 4.000000000000000000 ) ) ;
#4603=VERTEX_POINT ( 'NONE', #5005 ) ;
#4612=ADVANCED_FACE ( 'NONE', ( #10851 ), #5733, .F. ) ;
#4618=CARTESIAN_POINT ( 'NONE',  ( 80.00000000000001421, -74.24929059928631148, -32.00000000000000000 ) ) ;
#4619=DIRECTION ( 'NONE',  ( -0.000000000000000000, 1.000000000000000000, -1.927470528863119788E-16 ) ) ;
#4622=CARTESIAN_POINT ( 'NONE',  ( 80.00000000000001421, -76.24929059928631148, -4.000000000000000000 ) ) ;
#4665=VERTEX_POINT ( 'NONE', #4313 ) ;
#4689=ORIENTED_EDGE ( 'NONE', *, *, #6317, .F. ) ;
#4693=PRODUCT_DEFINITION_SHAPE ( 'NONE', 'NONE',  #11824 ) ;
#4699=DIRECTION ( 'NONE',  ( 0.000000000000000000, 0.000000000000000000, 1.000000000000000000 ) ) ;
#4714=LINE ( 'NONE', #9414, #13176 ) ;
#4725=ORIENTED_EDGE ( 'NONE', *, *, #15129, .T. ) ;
#4726=ADVANCED_FACE ( 'NONE', ( #1008 ), #5491, .F. ) ;
#4733=DIRECTION ( 'NONE',  ( -0.000000000000000000, 1.000000000000000000, 1.445602896647339163E-16 ) ) ;
#4735=VECTOR ( 'NONE', #1584, 1000.000000000000000 ) ;
#4787=CARTESIAN_POINT ( 'NONE',  ( 65.00000000000001421, -85.24929059928631148, 19.99999999999999645 ) ) ;
#4805=ORIENTED_EDGE ( 'NONE', *, *, #1604, .F. ) ;
#4817=FACE_BOUND ( 'NONE', #12208, .T. ) ;
#4829=AXIS2_PLACEMENT_3D ( 'NONE', #2380, #9392, #10464 ) ;
#4830=EDGE_LOOP ( 'NONE', ( #6439, #3846, #717, #747 ) ) ;
#4844=ADVANCED_FACE ( 'NONE', ( #3784 ), #15178, .F. ) ;
#4852=CIRCLE ( 'NONE', #8758, 2.500000000000002220 ) ;
#4853=LINE ( 'NONE', #2471, #10902 ) ;
#4856=AXIS2_PLACEMENT_3D ( 'NONE', #2110, #9126, #13810 ) ;
#4908=CARTESIAN_POINT ( 'NONE',  ( -65.00000000000001421, -85.27429059928628874, -19.99999999999999645 ) ) ;
#4911=EDGE_LOOP ( 'NONE', ( #15173, #5766, #7027, #12143 ) ) ;
#4913=CARTESIAN_POINT ( 'NONE',  ( 80.00000000000001421, -85.24929059928629727, -8.000000000000001776 ) ) ;
#4936=CARTESIAN_POINT ( 'NONE',  ( -80.00000000000001421, -72.24929059928631148, -34.99999999999999289 ) ) ;
#4937=CARTESIAN_POINT ( 'NONE',  ( 65.00000000000001421, -85.24929059928629727, -19.99999999999999645 ) ) ;
#4949=VECTOR ( 'NONE', #14665, 1000.000000000000000 ) ;
#4951=ADVANCED_FACE ( 'NONE', ( #2845 ), #608, .F. ) ;
#4958=( NAMED_UNIT ( * ) SI_UNIT ( $, .STERADIAN. ) SOLID_ANGLE_UNIT ( ) );
#4960=CARTESIAN_POINT ( 'NONE',  ( -65.00000000000001421, -85.27429059928630295, 19.99999999999999645 ) ) ;
#4967=EDGE_CURVE ( 'NONE', #1918, #3601, #12349, .T. ) ;
#4981=EDGE_LOOP ( 'NONE', ( #9685, #10145, #6681, #8940 ) ) ;
#4995=CARTESIAN_POINT ( 'NONE',  ( 65.00000000000001421, -87.24929059928631148, 17.50000000000000000 ) ) ;
#5005=CARTESIAN_POINT ( 'NONE',  ( -80.00000000000001421, -85.24929059928631148, -6.000000000000001776 ) ) ;
#5010=DIRECTION ( 'NONE',  ( -0.000000000000000000, 1.000000000000000000, 1.445602896647339163E-16 ) ) ;
#5040=EDGE_CURVE ( 'NONE', #3737, #14173, #9726, .T. ) ;
#5047=DIRECTION ( 'NONE',  ( 0.000000000000000000, -1.000000000000000000, 0.000000000000000000 ) ) ;
#5055=FACE_OUTER_BOUND ( 'NONE', #186, .T. ) ;
#5059=FACE_OUTER_BOUND ( 'NONE', #14115, .T. ) ;
#5060=DIRECTION ( 'NONE',  ( -1.000000000000000000, -0.000000000000000000, -0.000000000000000000 ) ) ;
#5065=CARTESIAN_POINT ( 'NONE',  ( 80.00000000000001421, -76.24929059928631148, 6.000000000000000000 ) ) ;
#5079=LINE ( 'NONE', #14471, #14346 ) ;
#5123=LINE ( 'NONE', #9825, #9641 ) ;
#5126=VERTEX_POINT ( 'NONE', #4380 ) ;
#5132=CARTESIAN_POINT ( 'NONE',  ( -65.00000000000001421, -87.24929059928631148, -19.99999999999999645 ) ) ;
#5136=EDGE_CURVE ( 'NONE', #6626, #4096, #6759, .T. ) ;
#5138=CARTESIAN_POINT ( 'NONE',  ( 80.00000000000001421, -85.24929059928629727, 8.000000000000001776 ) ) ;
#5156=ORIENTED_EDGE ( 'NONE', *, *, #3068, .F. ) ;
#5159=EDGE_LOOP ( 'NONE', ( #979, #8993, #2751, #12606 ) ) ;
#5165=LINE ( 'NONE', #9870, #11938 ) ;
#5173=DIRECTION ( 'NONE',  ( -1.000000000000000000, -0.000000000000000000, -0.000000000000000000 ) ) ;
#5202=DIRECTION ( 'NONE',  ( -0.000000000000000000, 1.000000000000000000, 1.445602896647339163E-16 ) ) ;
#5232=EDGE_LOOP ( 'NONE', ( #8647, #5473, #4214, #726 ) ) ;
#5235=CIRCLE ( 'NONE', #13834, 2.499999999999995115 ) ;
#5246=CIRCLE ( 'NONE', #566, 2.500000000000002220 ) ;
#5248=DIRECTION ( 'NONE',  ( -0.000000000000000000, 1.000000000000000000, 1.445602896647339163E-16 ) ) ;
#5251=LINE ( 'NONE', #3161, #1471 ) ;
#5258=CARTESIAN_POINT ( 'NONE',  ( -80.00000000000001421, -72.24929059928631148, 32.99999999999999289 ) ) ;
#5268=ORIENTED_EDGE ( 'NONE', *, *, #11010, .F. ) ;
#5281=DIRECTION ( 'NONE',  ( -0.000000000000000000, 0.000000000000000000, 1.000000000000000000 ) ) ;
#5298=CLOSED_SHELL ( 'NONE', ( #2279, #8838, #205, #2310, #158, #989, #295, #14342, #4726, #9925, #6833, #5770, #3240, #10021, #8792, #4218, #9347, #11590, #466, #841, #10171, #11159, #2355, #5808, #13395, #8012, #1329, #4951, #6597, #4844, #595, #13870, #1407, #14473, #19, #4612, #10820, #8389, #4033, #9757, #7954, #11082 ) ) ;
#5306=ORIENTED_EDGE ( 'NONE', *, *, #292, .T. ) ;
#5338=ORIENTED_EDGE ( 'NONE', *, *, #6398, .F. ) ;
#5341=VECTOR ( 'NONE', #11655, 1000.000000000000000 ) ;
#5343=FACE_OUTER_BOUND ( 'NONE', #8038, .T. ) ;
#5360=DIRECTION ( 'NONE',  ( -0.000000000000000000, 1.000000000000000000, 1.445602896647339163E-16 ) ) ;
#5385=LINE ( 'NONE', #12309, #6442 ) ;
#5410=AXIS2_PLACEMENT_3D ( 'NONE', #732, #590, #13668 ) ;
#5431=CARTESIAN_POINT ( 'NONE',  ( 80.00000000000001421, -74.24929059928631148, 32.99999999999999289 ) ) ;
#5441=VECTOR ( 'NONE', #1465, 1000.000000000000000 ) ;
#5442=CIRCLE ( 'NONE', #3961, 2.524999999999999467 ) ;
#5445=LINE ( 'NONE', #10142, #784 ) ;
#5459=EDGE_CURVE ( 'NONE', #12204, #404, #13672, .T. ) ;
#5463=EDGE_CURVE ( 'NONE', #14822, #2753, #9988, .T. ) ;
#5473=ORIENTED_EDGE ( 'NONE', *, *, #3106, .F. ) ;
#5474=DIRECTION ( 'NONE',  ( -0.000000000000000000, -0.000000000000000000, -1.000000000000000000 ) ) ;
#5476=VECTOR ( 'NONE', #606, 1000.000000000000000 ) ;
#5491=PLANE ( 'NONE',  #13564 ) ;
#5512=EDGE_CURVE ( 'NONE', #12689, #1978, #13829, .T. ) ;
#5529=DIRECTION ( 'NONE',  ( -0.000000000000000000, 1.734723475976817547E-15, 1.000000000000000000 ) ) ;
#5532=CARTESIAN_POINT ( 'NONE',  ( 65.00000000000001421, -85.24929059928631148, 17.47499999999999787 ) ) ;
#5548=DIRECTION ( 'NONE',  ( 1.000000000000000000, 0.000000000000000000, 0.000000000000000000 ) ) ;
#5564=EDGE_CURVE ( 'NONE', #5126, #12443, #5445, .T. ) ;
#5581=VECTOR ( 'NONE', #10295, 1000.000000000000000 ) ;
#5593=VERTEX_POINT ( 'NONE', #11673 ) ;
#5596=VERTEX_POINT ( 'NONE', #14145 ) ;
#5628=FACE_OUTER_BOUND ( 'NONE', #8055, .T. ) ;
#5658=EDGE_CURVE ( 'NONE', #5708, #81, #1209, .T. ) ;
#5666=DIRECTION ( 'NONE',  ( -0.000000000000000000, 1.000000000000000000, 1.445602896647339163E-16 ) ) ;
#5680=VECTOR ( 'NONE', #13405, 1000.000000000000000 ) ;
#5695=CARTESIAN_POINT ( 'NONE',  ( 65.00000000000001421, -85.27429059928630295, 19.99999999999999645 ) ) ;
#5699=VECTOR ( 'NONE', #5047, 1000.000000000000000 ) ;
#5701=CARTESIAN_POINT ( 'NONE',  ( -65.00000000000001421, -85.24929059928629727, -22.52499999999999503 ) ) ;
#5708=VERTEX_POINT ( 'NONE', #9608 ) ;
#5709=DIRECTION ( 'NONE',  ( 0.000000000000000000, 0.000000000000000000, -1.000000000000000000 ) ) ;
#5710=DIRECTION ( 'NONE',  ( -1.000000000000000000, -0.000000000000000000, -0.000000000000000000 ) ) ;
#5727=DIRECTION ( 'NONE',  ( 0.000000000000000000, -4.625929269271485914E-16, 1.000000000000000000 ) ) ;
#5733=CONICAL_SURFACE ( 'NONE', #9405, 2.524999999999999467, 0.7853981633973787790 ) ;
#5742=ORIENTED_EDGE ( 'NONE', *, *, #2357, .F. ) ;
#5766=ORIENTED_EDGE ( 'NONE', *, *, #4168, .F. ) ;
#5770=ADVANCED_FACE ( 'NONE', ( #5055 ), #1589, .F. ) ;
#5774=CARTESIAN_POINT ( 'NONE',  ( 80.00000000000001421, -72.24929059928631148, 32.99999999999999289 ) ) ;
#5777=ORIENTED_EDGE ( 'NONE', *, *, #9548, .F. ) ;
#5778=DIRECTION ( 'NONE',  ( -0.000000000000000000, 1.000000000000000000, 1.445602896647339163E-16 ) ) ;
#5808=ADVANCED_FACE ( 'NONE', ( #8588 ), #11973, .F. ) ;
#5816=CARTESIAN_POINT ( 'NONE',  ( 65.00000000000001421, -85.27429059928630295, 17.49999999999999645 ) ) ;
#5836=DIRECTION ( 'NONE',  ( -0.000000000000000000, 1.000000000000000000, 1.445602896647339163E-16 ) ) ;
#5838=DIRECTION ( 'NONE',  ( -0.000000000000000000, 1.000000000000000000, -0.000000000000000000 ) ) ;
#5865=LINE ( 'NONE', #5934, #7423 ) ;
#5878=DIRECTION ( 'NONE',  ( 0.000000000000000000, 0.000000000000000000, 1.000000000000000000 ) ) ;
#5890=DIRECTION ( 'NONE',  ( 0.000000000000000000, 0.000000000000000000, 1.000000000000000000 ) ) ;
#5906=LINE ( 'NONE', #11809, #1800 ) ;
#5934=CARTESIAN_POINT ( 'NONE',  ( -80.00000000000001421, -87.24929059928631148, -35.00000000000000000 ) ) ;
#5935=PRODUCT ( 'Bench-Mounted Base Unit', 'Bench-Mounted Base Unit', '', ( #9939 ) ) ;
#5941=CARTESIAN_POINT ( 'NONE',  ( -80.00000000000001421, -72.24929059928631148, -32.99999999999999289 ) ) ;
#5963=EDGE_CURVE ( 'NONE', #11368, #307, #12551, .T. ) ;
#5967=ORIENTED_EDGE ( 'NONE', *, *, #12555, .T. ) ;
#5991=LINE ( 'NONE', #13982, #7682 ) ;
#6017=DIRECTION ( 'NONE',  ( 0.000000000000000000, 0.7071067811865965336, 0.7071067811864985009 ) ) ;
#6047=DIRECTION ( 'NONE',  ( -0.000000000000000000, 1.000000000000000000, 1.445602896647339163E-16 ) ) ;
#6093=DIRECTION ( 'NONE',  ( -0.000000000000000000, 1.000000000000000000, 1.445602896647339163E-16 ) ) ;
#6103=CARTESIAN_POINT ( 'NONE',  ( -65.00000000000001421, -85.24929059928631148, 19.99999999999999645 ) ) ;
#6110=VECTOR ( 'NONE', #10667, 1000.000000000000000 ) ;
#6118=( LENGTH_UNIT ( ) NAMED_UNIT ( * ) SI_UNIT ( .MILLI., .METRE. ) );
#6136=LINE ( 'NONE', #13414, #13315 ) ;
#6144=CARTESIAN_POINT ( 'NONE',  ( 80.00000000000001421, -74.24929059928631148, 8.000000000000001776 ) ) ;
#6167=ORIENTED_EDGE ( 'NONE', *, *, #737, .T. ) ;
#6168=LINE ( 'NONE', #10855, #3858 ) ;
#6197=DIRECTION ( 'NONE',  ( 0.000000000000000000, -1.000000000000000000, 0.000000000000000000 ) ) ;
#6218=ORIENTED_EDGE ( 'NONE', *, *, #6317, .T. ) ;
#6220=DIRECTION ( 'NONE',  ( 0.000000000000000000, -0.000000000000000000, -1.000000000000000000 ) ) ;
#6244=EDGE_CURVE ( 'NONE', #1918, #8897, #3622, .T. ) ;
#6256=DIRECTION ( 'NONE',  ( -1.000000000000000000, -0.000000000000000000, -0.000000000000000000 ) ) ;
#6257=ORIENTED_EDGE ( 'NONE', *, *, #14806, .T. ) ;
#6273=EDGE_CURVE ( 'NONE', #4096, #3011, #4507, .T. ) ;
#6285=EDGE_CURVE ( 'NONE', #3011, #4096, #7215, .T. ) ;
#6309=EDGE_CURVE ( 'NONE', #12860, #6626, #5079, .T. ) ;
#6315=AXIS2_PLACEMENT_3D ( 'NONE', #4082, #8567, #11096 ) ;
#6317=EDGE_CURVE ( 'NONE', #5708, #9131, #4853, .T. ) ;
#6333=VECTOR ( 'NONE', #13403, 1000.000000000000000 ) ;
#6336=FACE_OUTER_BOUND ( 'NONE', #5159, .T. ) ;
#6343=CARTESIAN_POINT ( 'NONE',  ( -80.00000000000001421, -74.24929059928631148, 32.99999999999999289 ) ) ;
#6359=CARTESIAN_POINT ( 'NONE',  ( 80.00000000000001421, -74.24929059928631148, -32.99999999999999289 ) ) ;
#6363=ORIENTED_EDGE ( 'NONE', *, *, #7910, .F. ) ;
#6373=CARTESIAN_POINT ( 'NONE',  ( 65.00000000000001421, -85.24929059928629727, -17.47499999999999787 ) ) ;
#6379=LINE ( 'NONE', #3837, #7588 ) ;
#6382=ORIENTED_EDGE ( 'NONE', *, *, #13432, .F. ) ;
#6384=EDGE_LOOP ( 'NONE', ( #3018, #13555, #8675, #14447 ) ) ;
#6398=EDGE_CURVE ( 'NONE', #3110, #5708, #8832, .T. ) ;
#6424=DIRECTION ( 'NONE',  ( 0.000000000000000000, -1.000000000000000000, -1.445602896647339410E-16 ) ) ;
#6430=MECHANICAL_DESIGN_GEOMETRIC_PRESENTATION_REPRESENTATION('',(#11103),#8173);
#6439=ORIENTED_EDGE ( 'NONE', *, *, #11630, .F. ) ;
#6442=VECTOR ( 'NONE', #9938, 1000.000000000000000 ) ;
#6482=DIRECTION ( 'NONE',  ( 0.000000000000000000, 1.000000000000000000, 0.000000000000000000 ) ) ;
#6491=ORIENTED_EDGE ( 'NONE', *, *, #292, .F. ) ;
#6508=ORIENTED_EDGE ( 'NONE', *, *, #5564, .T. ) ;
#6515=ORIENTED_EDGE ( 'NONE', *, *, #4967, .T. ) ;
#6547=CARTESIAN_POINT ( 'NONE',  ( 80.00000000000001421, -74.24929059928631148, -4.000000000000000000 ) ) ;
#6569=FACE_BOUND ( 'NONE', #14058, .T. ) ;
#6572=EDGE_CURVE ( 'NONE', #4603, #341, #14994, .T. ) ;
#6581=CARTESIAN_POINT ( 'NONE',  ( 80.00000000000001421, -72.24929059928631148, 32.99999999999999289 ) ) ;
#6586=DIRECTION ( 'NONE',  ( 0.000000000000000000, 0.000000000000000000, 1.000000000000000000 ) ) ;
#6593=EDGE_LOOP ( 'NONE', ( #8805, #14552, #12286, #10579 ) ) ;
#6595=DIRECTION ( 'NONE',  ( 0.000000000000000000, 0.000000000000000000, 1.000000000000000000 ) ) ;
#6597=ADVANCED_FACE ( 'NONE', ( #3372 ), #13993, .F. ) ;
#6601=CYLINDRICAL_SURFACE ( 'NONE', #14097, 2.499999999999995115 ) ;
#6626=VERTEX_POINT ( 'NONE', #14226 ) ;
#6644=CARTESIAN_POINT ( 'NONE',  ( -65.00000000000001421, -87.24929059928631148, -22.49999999999999289 ) ) ;
#6649=VECTOR ( 'NONE', #3066, 1000.000000000000000 ) ;
#6679=ORIENTED_EDGE ( 'NONE', *, *, #10557, .F. ) ;
#6681=ORIENTED_EDGE ( 'NONE', *, *, #14568, .F. ) ;
#6682=CIRCLE ( 'NONE', #2012, 2.499999999999995115 ) ;
#6689=DIRECTION ( 'NONE',  ( 8.659560562354330119E-17, 0.7071067811865966446, -0.7071067811864982788 ) ) ;
#6693=PLANE ( 'NONE',  #1745 ) ;
#6727=APPLICATION_CONTEXT ( 'automotive_design' ) ;
#6733=DIRECTION ( 'NONE',  ( 0.000000000000000000, 0.000000000000000000, 1.000000000000000000 ) ) ;
#6759=LINE ( 'NONE', #5701, #8907 ) ;
#6789=FACE_OUTER_BOUND ( 'NONE', #12198, .T. ) ;
#6790=EDGE_CURVE ( 'NONE', #8699, #13251, #13959, .T. ) ;
#6833=ADVANCED_FACE ( 'NONE', ( #1880 ), #12202, .F. ) ;
#6840=DIRECTION ( 'NONE',  ( 0.000000000000000000, -1.445602896647339163E-16, 1.000000000000000000 ) ) ;
#6869=VECTOR ( 'NONE', #6197, 1000.000000000000000 ) ;
#6879=ORIENTED_EDGE ( 'NONE', *, *, #1296, .T. ) ;
#6884=EDGE_CURVE ( 'NONE', #1311, #12875, #671, .T. ) ;
#6885=CARTESIAN_POINT ( 'NONE',  ( 80.00000000000001421, -85.24929059928631148, 6.000000000000001776 ) ) ;
#6896=VERTEX_POINT ( 'NONE', #10051 ) ;
#6900=AXIS2_PLACEMENT_3D ( 'NONE', #9675, #14363, #13200 ) ;
#6908=EDGE_CURVE ( 'NONE', #3756, #9345, #14659, .T. ) ;
#6921=VERTEX_POINT ( 'NONE', #7514 ) ;
#6922=VECTOR ( 'NONE', #12220, 1000.000000000000000 ) ;
#6957=ORIENTED_EDGE ( 'NONE', *, *, #10179, .T. ) ;
#6959=ORIENTED_EDGE ( 'NONE', *, *, #4471, .T. ) ;
#6975=ORIENTED_EDGE ( 'NONE', *, *, #11701, .T. ) ;
#6977=CARTESIAN_POINT ( 'NONE',  ( 65.00000000000001421, -85.24929059928629727, -19.99999999999999645 ) ) ;
#6999=ORIENTED_EDGE ( 'NONE', *, *, #6309, .F. ) ;
#7005=EDGE_LOOP ( 'NONE', ( #7278, #13914, #3121, #1042 ) ) ;
#7006=CARTESIAN_POINT ( 'NONE',  ( -80.00000000000001421, -85.24929059928629727, -32.00000000000000000 ) ) ;
#7007=FACE_OUTER_BOUND ( 'NONE', #4325, .T. ) ;
#7010=ORIENTED_EDGE ( 'NONE', *, *, #570, .F. ) ;
#7024=CARTESIAN_POINT ( 'NONE',  ( 80.00000000000001421, -74.24929059928631148, -32.00000000000000000 ) ) ;
#7027=ORIENTED_EDGE ( 'NONE', *, *, #12056, .F. ) ;
#7047=PRODUCT_DEFINITION_CONTEXT ( 'detailed design', #6727, 'design' ) ;
#7063=AXIS2_PLACEMENT_3D ( 'NONE', #10433, #5666, #9206 ) ;
#7087=ORIENTED_EDGE ( 'NONE', *, *, #14806, .F. ) ;
#7088=AXIS2_PLACEMENT_3D ( 'NONE', #4212, #3992, #13456 ) ;
#7091=CARTESIAN_POINT ( 'NONE',  ( -65.00000000000001421, -85.24929059928629727, -19.99999999999999645 ) ) ;
#7119=CARTESIAN_POINT ( 'NONE',  ( -65.00000000000001421, -85.24929059928629727, -22.52499999999999503 ) ) ;
#7122=EDGE_CURVE ( 'NONE', #14307, #12689, #50, .T. ) ;
#7136=CARTESIAN_POINT ( 'NONE',  ( 80.00000000000001421, -72.24929059928631148, -32.99999999999999289 ) ) ;
#7158=CIRCLE ( 'NONE', #6900, 2.499999999999995115 ) ;
#7174=CARTESIAN_POINT ( 'NONE',  ( -65.00000000000001421, -85.27429059928628874, -19.99999999999999645 ) ) ;
#7207=ORIENTED_EDGE ( 'NONE', *, *, #4240, .T. ) ;
#7215=CIRCLE ( 'NONE', #3775, 2.524999999999999467 ) ;
#7232=LINE ( 'NONE', #11994, #12338 ) ;
#7240=ORIENTED_EDGE ( 'NONE', *, *, #1237, .T. ) ;
#7278=ORIENTED_EDGE ( 'NONE', *, *, #13558, .T. ) ;
#7297=EDGE_LOOP ( 'NONE', ( #10654, #11777, #11698, #13745 ) ) ;
#7300=EDGE_LOOP ( 'NONE', ( #831, #4689, #5338, #699 ) ) ;
#7326=CARTESIAN_POINT ( 'NONE',  ( 80.00000000000001421, -85.24929059928631148, -6.000000000000001776 ) ) ;
#7338=AXIS2_PLACEMENT_3D ( 'NONE', #917, #8086, #4699 ) ;
#7361=PLANE ( 'NONE',  #7545 ) ;
#7388=ORIENTED_EDGE ( 'NONE', *, *, #12717, .T. ) ;
#7399=SHAPE_DEFINITION_REPRESENTATION ( #4693, #11466 ) ;
#7423=VECTOR ( 'NONE', #10621, 1000.000000000000000 ) ;
#7424=VECTOR ( 'NONE', #6017, 1000.000000000000000 ) ;
#7460=ORIENTED_EDGE ( 'NONE', *, *, #5963, .F. ) ;
#7494=CARTESIAN_POINT ( 'NONE',  ( -80.00000000000001421, -85.24929059928629727, -8.000000000000001776 ) ) ;
#7495=DIRECTION ( 'NONE',  ( -0.000000000000000000, 1.000000000000000000, -1.927470528863119788E-16 ) ) ;
#7499=EDGE_CURVE ( 'NONE', #12860, #11933, #1183, .T. ) ;
#7504=CARTESIAN_POINT ( 'NONE',  ( 65.00000000000001421, -85.24929059928629727, -22.52499999999999503 ) ) ;
#7510=VECTOR ( 'NONE', #12955, 1000.000000000000000 ) ;
#7511=DIRECTION ( 'NONE',  ( 0.000000000000000000, 0.000000000000000000, 1.000000000000000000 ) ) ;
#7512=DIRECTION ( 'NONE',  ( 0.000000000000000000, 1.000000000000000000, 0.000000000000000000 ) ) ;
#7514=CARTESIAN_POINT ( 'NONE',  ( 80.00000000000001421, -85.24929059928631148, -6.000000000000001776 ) ) ;
#7519=ORIENTED_EDGE ( 'NONE', *, *, #12555, .F. ) ;
#7531=CONICAL_SURFACE ( 'NONE', #10770, 2.524999999999999467, 0.7853981633973787790 ) ;
#7532=AXIS2_PLACEMENT_3D ( 'NONE', #2290, #5836, #8060 ) ;
#7545=AXIS2_PLACEMENT_3D ( 'NONE', #7136, #11820, #6220 ) ;
#7559=CARTESIAN_POINT ( 'NONE',  ( -80.00000000000001421, -74.24929059928631148, 4.000000000000000000 ) ) ;
#7563=VECTOR ( 'NONE', #1330, 1000.000000000000000 ) ;
#7576=DIRECTION ( 'NONE',  ( -0.000000000000000000, -0.000000000000000000, 1.000000000000000000 ) ) ;
#7578=CARTESIAN_POINT ( 'NONE',  ( -80.00000000000001421, -85.24929059928629727, 32.00000000000000000 ) ) ;
#7588=VECTOR ( 'NONE', #14537, 1000.000000000000000 ) ;
#7590=DIRECTION ( 'NONE',  ( -1.000000000000000000, 0.000000000000000000, -0.000000000000000000 ) ) ;
#7592=ORIENTED_EDGE ( 'NONE', *, *, #395, .F. ) ;
#7607=VECTOR ( 'NONE', #2060, 1000.000000000000114 ) ;
#7641=CARTESIAN_POINT ( 'NONE',  ( -80.00000000000001421, -87.24929059928631148, -35.00000000000000000 ) ) ;
#7663=FACE_OUTER_BOUND ( 'NONE', #12595, .T. ) ;
#7668=AXIS2_PLACEMENT_3D ( 'NONE', #14426, #13271, #2720 ) ;
#7674=LINE ( 'NONE', #5065, #4949 ) ;
#7675=EDGE_LOOP ( 'NONE', ( #224, #12363, #13230, #10189, #4725, #12188, #13134, #11763, #6957, #12084, #12574, #3681, #7207, #4164, #14006, #13960, #1758, #14741, #98, #11796, #12384, #9778, #9830, #5306 ) ) ;
#7682=VECTOR ( 'NONE', #9367, 1000.000000000000000 ) ;
#7683=AXIS2_PLACEMENT_3D ( 'NONE', #14481, #1696, #13538 ) ;
#7685=ORIENTED_EDGE ( 'NONE', *, *, #3022, .T. ) ;
#7690=EDGE_LOOP ( 'NONE', ( #9118, #14926, #14895, #13440 ) ) ;
#7720=VERTEX_POINT ( 'NONE', #4913 ) ;
#7762=FACE_OUTER_BOUND ( 'NONE', #6384, .T. ) ;
#7778=CARTESIAN_POINT ( 'NONE',  ( 65.00000000000001421, -85.24929059928631148, 19.99999999999999645 ) ) ;
#7789=DIRECTION ( 'NONE',  ( 0.000000000000000000, 0.000000000000000000, 1.000000000000000000 ) ) ;
#7803=VERTEX_POINT ( 'NONE', #2677 ) ;
#7832=LINE ( 'NONE', #9986, #8019 ) ;
#7867=VERTEX_POINT ( 'NONE', #507 ) ;
#7869=PLANE ( 'NONE',  #11271 ) ;
#7884=CARTESIAN_POINT ( 'NONE',  ( 65.00000000000001421, -85.24929059928631148, 22.52499999999999503 ) ) ;
#7885=ORIENTED_EDGE ( 'NONE', *, *, #3435, .T. ) ;
#7894=FACE_OUTER_BOUND ( 'NONE', #7675, .T. ) ;
#7896=ORIENTED_EDGE ( 'NONE', *, *, #14591, .T. ) ;
#7910=EDGE_CURVE ( 'NONE', #14077, #15028, #4852, .T. ) ;
#7939=EDGE_LOOP ( 'NONE', ( #6975, #5742, #9609, #2491 ) ) ;
#7954=ADVANCED_FACE ( 'NONE', ( #7978 ), #960, .F. ) ;
#7956=LINE ( 'NONE', #935, #1937 ) ;
#7966=VERTEX_POINT ( 'NONE', #2202 ) ;
#7972=LINE ( 'NONE', #13736, #5341 ) ;
#7978=FACE_OUTER_BOUND ( 'NONE', #8473, .T. ) ;
#8006=LINE ( 'NONE', #11533, #9635 ) ;
#8012=ADVANCED_FACE ( 'NONE', ( #4817, #13206, #11743 ), #8218, .F. ) ;
#8019=VECTOR ( 'NONE', #733, 1000.000000000000000 ) ;
#8023=DIRECTION ( 'NONE',  ( -1.000000000000000000, -0.000000000000000000, -0.000000000000000000 ) ) ;
#8038=EDGE_LOOP ( 'NONE', ( #14697, #11754, #6491, #3809 ) ) ;
#8045=FACE_OUTER_BOUND ( 'NONE', #6593, .T. ) ;
#8050=CONICAL_SURFACE ( 'NONE', #7063, 2.524999999999999467, 0.7853981633973787790 ) ;
#8055=EDGE_LOOP ( 'NONE', ( #521, #605, #2938, #2698 ) ) ;
#8060=DIRECTION ( 'NONE',  ( 0.000000000000000000, 0.000000000000000000, 1.000000000000000000 ) ) ;
#8084=ORIENTED_EDGE ( 'NONE', *, *, #12441, .F. ) ;
#8086=DIRECTION ( 'NONE',  ( -0.000000000000000000, 1.000000000000000000, 1.445602896647339163E-16 ) ) ;
#8092=ORIENTED_EDGE ( 'NONE', *, *, #12424, .T. ) ;
#8118=LINE ( 'NONE', #10660, #8442 ) ;
#8168=CARTESIAN_POINT ( 'NONE',  ( -65.00000000000001421, -85.24929059928629727, -19.99999999999999645 ) ) ;
#8173=( GEOMETRIC_REPRESENTATION_CONTEXT ( 3 ) GLOBAL_UNCERTAINTY_ASSIGNED_CONTEXT ( ( #2729 ) ) GLOBAL_UNIT_ASSIGNED_CONTEXT ( ( #6118, #13118, #1636 ) ) REPRESENTATION_CONTEXT ( 'NONE', 'WORKASPACE' ) );
#8205=LINE ( 'NONE', #2577, #1878 ) ;
#8218=PLANE ( 'NONE',  #177 ) ;
#8219=ORIENTED_EDGE ( 'NONE', *, *, #14946, .T. ) ;
#8246=ORIENTED_EDGE ( 'NONE', *, *, #3581, .F. ) ;
#8253=ORIENTED_EDGE ( 'NONE', *, *, #5136, .F. ) ;
#8259=ORIENTED_EDGE ( 'NONE', *, *, #5459, .T. ) ;
#8295=ORIENTED_EDGE ( 'NONE', *, *, #3022, .F. ) ;
#8317=AXIS2_PLACEMENT_3D ( 'NONE', #8808, #12426, #7511 ) ;
#8335=CYLINDRICAL_SURFACE ( 'NONE', #13080, 2.499999999999995115 ) ;
#8338=DIRECTION ( 'NONE',  ( 0.000000000000000000, 0.000000000000000000, 1.000000000000000000 ) ) ;
#8340=DIRECTION ( 'NONE',  ( -0.000000000000000000, 1.000000000000000000, 1.445602896647339163E-16 ) ) ;
#8377=DIRECTION ( 'NONE',  ( 0.000000000000000000, 1.000000000000000000, 0.000000000000000000 ) ) ;
#8389=ADVANCED_FACE ( 'NONE', ( #3794 ), #4159, .F. ) ;
#8414=DIRECTION ( 'NONE',  ( 0.000000000000000000, -1.000000000000000000, 0.000000000000000000 ) ) ;
#8415=DIRECTION ( 'NONE',  ( -0.000000000000000000, -0.000000000000000000, -1.000000000000000000 ) ) ;
#8420=VECTOR ( 'NONE', #7576, 1000.000000000000000 ) ;
#8442=VECTOR ( 'NONE', #190, 1000.000000000000000 ) ;
#8473=EDGE_LOOP ( 'NONE', ( #7460, #7519, #14460, #9754 ) ) ;
#8478=DIRECTION ( 'NONE',  ( 0.000000000000000000, -1.734723475976817547E-15, 1.000000000000000000 ) ) ;
#8490=FACE_OUTER_BOUND ( 'NONE', #7690, .T. ) ;
#8508=VECTOR ( 'NONE', #4245, 1000.000000000000000 ) ;
#8512=EDGE_CURVE ( 'NONE', #3697, #404, #13554, .T. ) ;
#8519=CIRCLE ( 'NONE', #10481, 2.524999999999999467 ) ;
#8566=LINE ( 'NONE', #3938, #2941 ) ;
#8567=DIRECTION ( 'NONE',  ( 0.000000000000000000, 0.000000000000000000, 1.000000000000000000 ) ) ;
#8570=EDGE_CURVE ( 'NONE', #538, #14822, #4236, .T. ) ;
#8584=DIRECTION ( 'NONE',  ( -1.000000000000000000, -0.000000000000000000, -0.000000000000000000 ) ) ;
#8588=FACE_OUTER_BOUND ( 'NONE', #10457, .T. ) ;
#8647=ORIENTED_EDGE ( 'NONE', *, *, #157, .T. ) ;
#8651=AXIS2_PLACEMENT_3D ( 'NONE', #5695, #5778, #14000 ) ;
#8656=ORIENTED_EDGE ( 'NONE', *, *, #14758, .F. ) ;
#8675=ORIENTED_EDGE ( 'NONE', *, *, #11630, .T. ) ;
#8699=VERTEX_POINT ( 'NONE', #4995 ) ;
#8702=CARTESIAN_POINT ( 'NONE',  ( 65.00000000000001421, -85.24929059928631148, 19.99999999999999645 ) ) ;
#8714=CARTESIAN_POINT ( 'NONE',  ( -80.00000000000001421, -85.24929059928629727, 8.000000000000001776 ) ) ;
#8723=DIRECTION ( 'NONE',  ( -0.000000000000000000, 1.445602896647339163E-16, 1.000000000000000000 ) ) ;
#8758=AXIS2_PLACEMENT_3D ( 'NONE', #14739, #5360, #11662 ) ;
#8791=CARTESIAN_POINT ( 'NONE',  ( -65.00000000000001421, -85.24929059928629727, -17.47499999999999787 ) ) ;
#8792=ADVANCED_FACE ( 'NONE', ( #9918 ), #8974, .F. ) ;
#8804=DIRECTION ( 'NONE',  ( 0.000000000000000000, 1.445602896647339410E-16, -1.000000000000000000 ) ) ;
#8805=ORIENTED_EDGE ( 'NONE', *, *, #12012, .F. ) ;
#8808=CARTESIAN_POINT ( 'NONE',  ( 65.00000000000001421, -85.24929059928631148, 19.99999999999999645 ) ) ;
#8810=PLANE ( 'NONE',  #11138 ) ;
#8827=VECTOR ( 'NONE', #1058, 1000.000000000000000 ) ;
#8832=LINE ( 'NONE', #13453, #12362 ) ;
#8838=ADVANCED_FACE ( 'NONE', ( #12287 ), #9984, .F. ) ;
#8845=CARTESIAN_POINT ( 'NONE',  ( 80.00000000000001421, -74.24929059928631148, 32.99999999999999289 ) ) ;
#8866=AXIS2_PLACEMENT_3D ( 'NONE', #2049, #11504, #6586 ) ;
#8883=AXIS2_PLACEMENT_3D ( 'NONE', #893, #13754, #6595 ) ;
#8889=DIRECTION ( 'NONE',  ( -1.000000000000000000, 0.000000000000000000, 0.000000000000000000 ) ) ;
#8897=VERTEX_POINT ( 'NONE', #3204 ) ;
#8907=VECTOR ( 'NONE', #6689, 1000.000000000000114 ) ;
#8908=DIRECTION ( 'NONE',  ( -0.000000000000000000, 1.000000000000000000, 1.445602896647339163E-16 ) ) ;
#8922=LINE ( 'NONE', #13692, #5476 ) ;
#8923=CARTESIAN_POINT ( 'NONE',  ( 80.00000000000001421, -74.24929059928631148, 8.000000000000001776 ) ) ;
#8940=ORIENTED_EDGE ( 'NONE', *, *, #4556, .T. ) ;
#8946=LINE ( 'NONE', #6343, #8508 ) ;
#8959=DIRECTION ( 'NONE',  ( -0.000000000000000000, 1.000000000000000000, 1.445602896647339163E-16 ) ) ;
#8961=PLANE ( 'NONE',  #9526 ) ;
#8971=ORIENTED_EDGE ( 'NONE', *, *, #1237, .F. ) ;
#8974=PLANE ( 'NONE',  #5410 ) ;
#8988=VECTOR ( 'NONE', #1480, 1000.000000000000000 ) ;
#8993=ORIENTED_EDGE ( 'NONE', *, *, #14534, .F. ) ;
#9002=LINE ( 'NONE', #15011, #3133 ) ;
#9005=DIRECTION ( 'NONE',  ( -0.000000000000000000, 1.000000000000000000, 1.445602896647339163E-16 ) ) ;
#9029=AXIS2_PLACEMENT_3D ( 'NONE', #3675, #8377, #3051 ) ;
#9053=DIRECTION ( 'NONE',  ( -0.000000000000000000, 1.000000000000000000, 1.445602896647339163E-16 ) ) ;
#9085=CARTESIAN_POINT ( 'NONE',  ( 65.00000000000001421, -85.27429059928628874, -22.50000000000000000 ) ) ;
#9087=LINE ( 'NONE', #2153, #475 ) ;
#9108=DIRECTION ( 'NONE',  ( -0.000000000000000000, -0.000000000000000000, 1.000000000000000000 ) ) ;
#9118=ORIENTED_EDGE ( 'NONE', *, *, #15142, .F. ) ;
#9126=DIRECTION ( 'NONE',  ( -0.000000000000000000, 1.000000000000000000, 1.445602896647339163E-16 ) ) ;
#9131=VERTEX_POINT ( 'NONE', #9191 ) ;
#9173=ORIENTED_EDGE ( 'NONE', *, *, #13799, .F. ) ;
#9180=DIRECTION ( 'NONE',  ( 0.000000000000000000, 0.7071067811865965336, 0.7071067811864985009 ) ) ;
#9191=CARTESIAN_POINT ( 'NONE',  ( -80.00000000000001421, -76.24929059928631148, 4.000000000000000000 ) ) ;
#9206=DIRECTION ( 'NONE',  ( 0.000000000000000000, 0.000000000000000000, 1.000000000000000000 ) ) ;
#9209=LINE ( 'NONE', #9513, #6110 ) ;
#9218=ORIENTED_EDGE ( 'NONE', *, *, #12034, .F. ) ;
#9233=ORIENTED_EDGE ( 'NONE', *, *, #11996, .F. ) ;
#9272=VERTEX_POINT ( 'NONE', #13957 ) ;
#9278=CARTESIAN_POINT ( 'NONE',  ( 80.00000000000001421, -74.24929059928631148, 4.000000000000000000 ) ) ;
#9288=EDGE_LOOP ( 'NONE', ( #2050, #8246, #5156, #237 ) ) ;
#9303=DIRECTION ( 'NONE',  ( 0.000000000000000000, 0.000000000000000000, 1.000000000000000000 ) ) ;
#9308=ORIENTED_EDGE ( 'NONE', *, *, #11666, .F. ) ;
#9321=VERTEX_POINT ( 'NONE', #1491 ) ;
#9328=EDGE_CURVE ( 'NONE', #4038, #10741, #8566, .T. ) ;
#9345=VERTEX_POINT ( 'NONE', #5258 ) ;
#9347=ADVANCED_FACE ( 'NONE', ( #6336 ), #7869, .F. ) ;
#9357=CARTESIAN_POINT ( 'NONE',  ( -80.00000000000001421, -85.24929059928629727, 8.000000000000001776 ) ) ;
#9367=DIRECTION ( 'NONE',  ( -0.000000000000000000, -1.000000000000000000, 4.625929269271485914E-16 ) ) ;
#9392=DIRECTION ( 'NONE',  ( 0.000000000000000000, 1.000000000000000000, 0.000000000000000000 ) ) ;
#9398=CARTESIAN_POINT ( 'NONE',  ( 80.00000000000001421, -76.24929059928631148, -6.000000000000000000 ) ) ;
#9399=DIRECTION ( 'NONE',  ( -0.000000000000000000, 1.000000000000000000, 1.445602896647339163E-16 ) ) ;
#9405=AXIS2_PLACEMENT_3D ( 'NONE', #313, #9711, #3835 ) ;
#9413=ORIENTED_EDGE ( 'NONE', *, *, #11907, .F. ) ;
#9414=CARTESIAN_POINT ( 'NONE',  ( -80.00000000000001421, -76.24929059928631148, 4.000000000000000000 ) ) ;
#9473=ORIENTED_EDGE ( 'NONE', *, *, #13825, .T. ) ;
#9478=ORIENTED_EDGE ( 'NONE', *, *, #9548, .T. ) ;
#9483=ORIENTED_EDGE ( 'NONE', *, *, #11943, .F. ) ;
#9490=CIRCLE ( 'NONE', #3334, 2.500000000000002220 ) ;
#9494=CARTESIAN_POINT ( 'NONE',  ( 80.00000000000001421, -74.24929059928631148, -4.000000000000000000 ) ) ;
#9513=CARTESIAN_POINT ( 'NONE',  ( 80.00000000000001421, -74.24929059928631148, -32.00000000000000000 ) ) ;
#9524=AXIS2_PLACEMENT_3D ( 'NONE', #4960, #6047, #10731 ) ;
#9526=AXIS2_PLACEMENT_3D ( 'NONE', #14805, #6424, #8804 ) ;
#9527=ORIENTED_EDGE ( 'NONE', *, *, #6285, .F. ) ;
#9536=AXIS2_PLACEMENT_3D ( 'NONE', #7778, #13704, #1919 ) ;
#9548=EDGE_CURVE ( 'NONE', #13009, #9321, #8519, .T. ) ;
#9559=DIRECTION ( 'NONE',  ( 0.000000000000000000, -4.625929269271485914E-16, -1.000000000000000000 ) ) ;
#9608=CARTESIAN_POINT ( 'NONE',  ( 80.00000000000001421, -76.24929059928631148, 4.000000000000000000 ) ) ;
#9609=ORIENTED_EDGE ( 'NONE', *, *, #5463, .F. ) ;
#9627=ORIENTED_EDGE ( 'NONE', *, *, #13050, .F. ) ;
#9635=VECTOR ( 'NONE', #5710, 1000.000000000000000 ) ;
#9636=CARTESIAN_POINT ( 'NONE',  ( 80.00000000000001421, -85.24929059928629727, 32.00000000000000000 ) ) ;
#9637=LINE ( 'NONE', #5941, #5441 ) ;
#9641=VECTOR ( 'NONE', #14506, 1000.000000000000000 ) ;
#9644=PLANE ( 'NONE',  #9653 ) ;
#9647=VECTOR ( 'NONE', #14126, 1000.000000000000000 ) ;
#9653=AXIS2_PLACEMENT_3D ( 'NONE', #2781, #167, #13318 ) ;
#9673=EDGE_CURVE ( 'NONE', #246, #531, #7832, .T. ) ;
#9675=CARTESIAN_POINT ( 'NONE',  ( -65.00000000000001421, -87.24929059928631148, 19.99999999999999645 ) ) ;
#9685=ORIENTED_EDGE ( 'NONE', *, *, #11666, .T. ) ;
#9697=CARTESIAN_POINT ( 'NONE',  ( 65.00000000000001421, -85.24929059928631148, 17.47499999999999787 ) ) ;
#9704=ORIENTED_EDGE ( 'NONE', *, *, #6908, .F. ) ;
#9711=DIRECTION ( 'NONE',  ( -0.000000000000000000, 1.000000000000000000, 1.445602896647339163E-16 ) ) ;
#9726=LINE ( 'NONE', #9869, #1285 ) ;
#9730=CARTESIAN_POINT ( 'NONE',  ( 80.00000000000001421, -74.24929059928631148, -8.000000000000001776 ) ) ;
#9743=LINE ( 'NONE', #2804, #1766 ) ;
#9749=ORIENTED_EDGE ( 'NONE', *, *, #5658, .F. ) ;
#9750=LINE ( 'NONE', #9896, #5699 ) ;
#9754=ORIENTED_EDGE ( 'NONE', *, *, #1430, .T. ) ;
#9757=ADVANCED_FACE ( 'NONE', ( #12841 ), #3602, .F. ) ;
#9778=ORIENTED_EDGE ( 'NONE', *, *, #3068, .T. ) ;
#9779=DIRECTION ( 'NONE',  ( 0.000000000000000000, -1.445602896647339163E-16, 1.000000000000000000 ) ) ;
#9788=CONICAL_SURFACE ( 'NONE', #9536, 2.524999999999999467, 0.7853981633973787790 ) ;
#9808=AXIS2_PLACEMENT_3D ( 'NONE', #7326, #3852, #13326 ) ;
#9825=CARTESIAN_POINT ( 'NONE',  ( 80.00000000000001421, -72.24929059928631148, 32.99999999999999289 ) ) ;
#9830=ORIENTED_EDGE ( 'NONE', *, *, #3711, .T. ) ;
#9836=DIRECTION ( 'NONE',  ( 0.000000000000000000, 0.000000000000000000, 1.000000000000000000 ) ) ;
#9869=CARTESIAN_POINT ( 'NONE',  ( 80.00000000000001421, -87.24929059928631148, -35.00000000000000000 ) ) ;
#9870=CARTESIAN_POINT ( 'NONE',  ( 80.00000000000001421, -85.24929059928631148, -6.000000000000001776 ) ) ;
#9896=CARTESIAN_POINT ( 'NONE',  ( 80.00000000000001421, -72.24929059928631148, -32.99999999999999289 ) ) ;
#9901=LINE ( 'NONE', #7578, #1038 ) ;
#9910=AXIS2_PLACEMENT_3D ( 'NONE', #6144, #10827, #288 ) ;
#9918=FACE_OUTER_BOUND ( 'NONE', #4981, .T. ) ;
#9922=CARTESIAN_POINT ( 'NONE',  ( 80.00000000000001421, -85.24929059928629727, 32.00000000000000000 ) ) ;
#9925=ADVANCED_FACE ( 'NONE', ( #13214 ), #7361, .F. ) ;
#9938=DIRECTION ( 'NONE',  ( 0.000000000000000000, 1.000000000000000000, 0.000000000000000000 ) ) ;
#9939=PRODUCT_CONTEXT ( 'NONE', #12966, 'mechanical' ) ;
#9984=CYLINDRICAL_SURFACE ( 'NONE', #725, 2.499999999999995115 ) ;
#9986=CARTESIAN_POINT ( 'NONE',  ( 80.00000000000001421, -74.24929059928631148, -8.000000000000001776 ) ) ;
#9988=LINE ( 'NONE', #2127, #13101 ) ;
#9994=VECTOR ( 'NONE', #11652, 1000.000000000000000 ) ;
#10008=DIRECTION ( 'NONE',  ( 0.000000000000000000, -1.000000000000000000, 1.734723475976817547E-15 ) ) ;
#10021=ADVANCED_FACE ( 'NONE', ( #6569, #10045, #638 ), #8961, .F. ) ;
#10044=LINE ( 'NONE', #2965, #2026 ) ;
#10045=FACE_BOUND ( 'NONE', #15042, .T. ) ;
#10051=CARTESIAN_POINT ( 'NONE',  ( -80.00000000000001421, -87.24929059928631148, 35.00000000000000000 ) ) ;
#10060=CARTESIAN_POINT ( 'NONE',  ( 65.00000000000001421, -85.24929059928629727, -19.99999999999999645 ) ) ;
#10073=DIRECTION ( 'NONE',  ( -0.000000000000000000, -0.000000000000000000, -1.000000000000000000 ) ) ;
#10076=ORIENTED_EDGE ( 'NONE', *, *, #11377, .F. ) ;
#10142=CARTESIAN_POINT ( 'NONE',  ( -80.00000000000001421, -74.24929059928631148, 32.00000000000000000 ) ) ;
#10145=ORIENTED_EDGE ( 'NONE', *, *, #9673, .F. ) ;
#10164=FACE_OUTER_BOUND ( 'NONE', #4137, .T. ) ;
#10171=ADVANCED_FACE ( 'NONE', ( #14880 ), #4332, .F. ) ;
#10179=EDGE_CURVE ( 'NONE', #1863, #2944, #2032, .T. ) ;
#10189=ORIENTED_EDGE ( 'NONE', *, *, #11036, .T. ) ;
#10194=DIRECTION ( 'NONE',  ( 0.000000000000000000, 0.000000000000000000, 1.000000000000000000 ) ) ;
#10228=ORIENTED_EDGE ( 'NONE', *, *, #11701, .F. ) ;
#10248=ORIENTED_EDGE ( 'NONE', *, *, #14140, .F. ) ;
#10249=CARTESIAN_POINT ( 'NONE',  ( 65.00000000000001421, -87.24929059928631148, 19.99999999999999645 ) ) ;
#10255=ORIENTED_EDGE ( 'NONE', *, *, #11943, .T. ) ;
#10277=CARTESIAN_POINT ( 'NONE',  ( 80.00000000000001421, -74.24929059928631148, -4.000000000000000000 ) ) ;
#10295=DIRECTION ( 'NONE',  ( -1.000000000000000000, -0.000000000000000000, -0.000000000000000000 ) ) ;
#10347=DIRECTION ( 'NONE',  ( -0.000000000000000000, 1.000000000000000000, 1.445602896647339163E-16 ) ) ;
#10353=FACE_OUTER_BOUND ( 'NONE', #4830, .T. ) ;
#10391=DIRECTION ( 'NONE',  ( -0.000000000000000000, -0.000000000000000000, 1.000000000000000000 ) ) ;
#10397=CYLINDRICAL_SURFACE ( 'NONE', #3656, 2.499999999999995115 ) ;
#10431=CARTESIAN_POINT ( 'NONE',  ( 65.00000000000001421, -85.27429059928628874, -19.99999999999999645 ) ) ;
#10433=CARTESIAN_POINT ( 'NONE',  ( -65.00000000000001421, -85.24929059928629727, -19.99999999999999645 ) ) ;
#10443=ORIENTED_EDGE ( 'NONE', *, *, #2601, .F. ) ;
#10457=EDGE_LOOP ( 'NONE', ( #12897, #10443, #12003, #10766 ) ) ;
#10464=DIRECTION ( 'NONE',  ( 0.000000000000000000, -0.000000000000000000, 1.000000000000000000 ) ) ;
#10468=LINE ( 'NONE', #15161, #15047 ) ;
#10471=LINE ( 'NONE', #4622, #12471 ) ;
#10481=AXIS2_PLACEMENT_3D ( 'NONE', #4937, #14253, #2322 ) ;
#10487=CARTESIAN_POINT ( 'NONE',  ( 65.00000000000001421, -85.24929059928629727, -19.99999999999999645 ) ) ;
#10557=EDGE_CURVE ( 'NONE', #6896, #2170, #13482, .T. ) ;
#10579=ORIENTED_EDGE ( 'NONE', *, *, #14361, .F. ) ;
#10609=ORIENTED_EDGE ( 'NONE', *, *, #11615, .F. ) ;
#10619=AXIS2_PLACEMENT_3D ( 'NONE', #3135, #8908, #12605 ) ;
#10621=DIRECTION ( 'NONE',  ( 0.000000000000000000, 1.000000000000000000, 4.625929269271485914E-16 ) ) ;
#10627=DIRECTION ( 'NONE',  ( 0.000000000000000000, 0.000000000000000000, 1.000000000000000000 ) ) ;
#10650=AXIS2_PLACEMENT_3D ( 'NONE', #6359, #13421, #13288 ) ;
#10654=ORIENTED_EDGE ( 'NONE', *, *, #8512, .T. ) ;
#10656=EDGE_LOOP ( 'NONE', ( #3306, #13997, #15212, #9478 ) ) ;
#10660=CARTESIAN_POINT ( 'NONE',  ( 80.00000000000001421, -74.24929059928631148, -32.99999999999999289 ) ) ;
#10667=DIRECTION ( 'NONE',  ( -1.000000000000000000, -0.000000000000000000, -0.000000000000000000 ) ) ;
#10687=ORIENTED_EDGE ( 'NONE', *, *, #6273, .F. ) ;
#10699=LINE ( 'NONE', #14089, #7424 ) ;
#10701=EDGE_CURVE ( 'NONE', #3972, #9345, #15026, .T. ) ;
#10707=ADVANCED_BREP_SHAPE_REPRESENTATION ( '', ( #14171, #6315 ), #3366 ) ;
#10709=ORIENTED_EDGE ( 'NONE', *, *, #11615, .T. ) ;
#10731=DIRECTION ( 'NONE',  ( 0.000000000000000000, 0.000000000000000000, 1.000000000000000000 ) ) ;
#10741=VERTEX_POINT ( 'NONE', #3322 ) ;
#10746=VECTOR ( 'NONE', #3659, 1000.000000000000000 ) ;
#10754=AXIS2_PLACEMENT_3D ( 'NONE', #5774, #15225, #824 ) ;
#10760=ORIENTED_EDGE ( 'NONE', *, *, #3385, .F. ) ;
#10766=ORIENTED_EDGE ( 'NONE', *, *, #11531, .T. ) ;
#10770=AXIS2_PLACEMENT_3D ( 'NONE', #13769, #12692, #4221 ) ;
#10798=LINE ( 'NONE', #11870, #7563 ) ;
#10799=PLANE ( 'NONE',  #3425 ) ;
#10820=ADVANCED_FACE ( 'NONE', ( #8490 ), #3636, .F. ) ;
#10821=DIRECTION ( 'NONE',  ( 0.000000000000000000, -1.000000000000000000, -1.927470528863119788E-16 ) ) ;
#10827=DIRECTION ( 'NONE',  ( 0.000000000000000000, -1.000000000000000000, 0.000000000000000000 ) ) ;
#10848=ORIENTED_EDGE ( 'NONE', *, *, #5512, .F. ) ;
#10851=FACE_OUTER_BOUND ( 'NONE', #3833, .T. ) ;
#10855=CARTESIAN_POINT ( 'NONE',  ( -80.00000000000001421, -74.24929059928631148, -32.99999999999999289 ) ) ;
#10857=DIRECTION ( 'NONE',  ( -0.000000000000000000, 1.000000000000000000, 1.445602896647339163E-16 ) ) ;
#10864=CIRCLE ( 'NONE', #10619, 2.500000000000002220 ) ;
#10878=AXIS2_PLACEMENT_3D ( 'NONE', #11329, #793, #10194 ) ;
#10887=CIRCLE ( 'NONE', #4479, 2.500000000000002220 ) ;
#10901=DIRECTION ( 'NONE',  ( 0.000000000000000000, -1.000000000000000000, 1.445602896647339410E-16 ) ) ;
#10902=VECTOR ( 'NONE', #1466, 1000.000000000000000 ) ;
#10983=CIRCLE ( 'NONE', #9524, 2.500000000000002220 ) ;
#10997=EDGE_LOOP ( 'NONE', ( #13335, #6679, #13516, #9218, #13346, #10228, #13724, #8656, #8295, #7010, #1752, #9233, #4243, #11364, #9173, #14001, #10248, #11008, #9308, #1389, #11581, #1245, #1615, #8084 ) ) ;
#11002=LINE ( 'NONE', #14678, #6649 ) ;
#11008=ORIENTED_EDGE ( 'NONE', *, *, #157, .F. ) ;
#11010=EDGE_CURVE ( 'NONE', #12204, #7720, #14766, .T. ) ;
#11014=EDGE_CURVE ( 'NONE', #81, #14307, #15002, .T. ) ;
#11031=DIRECTION ( 'NONE',  ( 0.000000000000000000, 1.000000000000000000, 0.000000000000000000 ) ) ;
#11036=EDGE_CURVE ( 'NONE', #1083, #12366, #13921, .T. ) ;
#11038=CARTESIAN_POINT ( 'NONE',  ( 65.00000000000001421, -85.24929059928631148, 22.49999999999999289 ) ) ;
#11039=LINE ( 'NONE', #494, #8420 ) ;
#11059=LINE ( 'NONE', #9922, #3599 ) ;
#11065=CARTESIAN_POINT ( 'NONE',  ( 80.00000000000001421, -87.24929059928631148, 35.00000000000000000 ) ) ;
#11079=DIRECTION ( 'NONE',  ( 0.000000000000000000, -1.734723475976817547E-15, -1.000000000000000000 ) ) ;
#11082=ADVANCED_FACE ( 'NONE', ( #13849 ), #7531, .F. ) ;
#11096=DIRECTION ( 'NONE',  ( 1.000000000000000000, 0.000000000000000000, 0.000000000000000000 ) ) ;
#11103=STYLED_ITEM('',(#15244),#14171);
#11138=AXIS2_PLACEMENT_3D ( 'NONE', #14735, #8889, #723 ) ;
#11139=LINE ( 'NONE', #6373, #13677 ) ;
#11142=VECTOR ( 'NONE', #12001, 1000.000000000000000 ) ;
#11149=DIRECTION ( 'NONE',  ( -0.000000000000000000, 1.000000000000000000, 1.445602896647339163E-16 ) ) ;
#11159=ADVANCED_FACE ( 'NONE', ( #3540 ), #1071, .F. ) ;
#11183=CARTESIAN_POINT ( 'NONE',  ( 80.00000000000001421, -87.24929059928631148, -35.00000000000000000 ) ) ;
#11244=DIRECTION ( 'NONE',  ( -1.000000000000000000, 0.000000000000000000, -0.000000000000000000 ) ) ;
#11271=AXIS2_PLACEMENT_3D ( 'NONE', #6547, #14942, #11244 ) ;
#11329=CARTESIAN_POINT ( 'NONE',  ( -65.00000000000001421, -85.24929059928631148, 19.99999999999999645 ) ) ;
#11343=DIRECTION ( 'NONE',  ( -0.000000000000000000, 1.000000000000000000, 1.445602896647339163E-16 ) ) ;
#11344=VECTOR ( 'NONE', #9180, 1000.000000000000000 ) ;
#11346=EDGE_LOOP ( 'NONE', ( #1722, #15106, #11595, #10255 ) ) ;
#11364=ORIENTED_EDGE ( 'NONE', *, *, #6572, .F. ) ;
#11368=VERTEX_POINT ( 'NONE', #13237 ) ;
#11377=EDGE_CURVE ( 'NONE', #4665, #13009, #11139, .T. ) ;
#11378=EDGE_CURVE ( 'NONE', #12689, #538, #11059, .T. ) ;
#11386=VECTOR ( 'NONE', #2054, 1000.000000000000000 ) ;
#11398=CARTESIAN_POINT ( 'NONE',  ( -80.00000000000001421, -74.24929059928631148, 4.000000000000000000 ) ) ;
#11420=VERTEX_POINT ( 'NONE', #2126 ) ;
#11454=DIRECTION ( 'NONE',  ( -1.000000000000000000, -0.000000000000000000, -0.000000000000000000 ) ) ;
#11466=SHAPE_REPRESENTATION ( 'Bench-Mounted Base Unit', ( #6315 ), #3366 ) ;
#11469=CARTESIAN_POINT ( 'NONE',  ( 80.00000000000001421, -87.24929059928631148, -35.00000000000000000 ) ) ;
#11471=AXIS2_PLACEMENT_3D ( 'NONE', #6977, #9053, #12831 ) ;
#11479=CYLINDRICAL_SURFACE ( 'NONE', #12079, 2.499999999999995115 ) ;
#11488=VECTOR ( 'NONE', #11633, 1000.000000000000000 ) ;
#11489=EDGE_LOOP ( 'NONE', ( #5967, #3959 ) ) ;
#11490=LINE ( 'NONE', #14804, #13814 ) ;
#11504=DIRECTION ( 'NONE',  ( -0.000000000000000000, 1.000000000000000000, 1.445602896647339163E-16 ) ) ;
#11508=CARTESIAN_POINT ( 'NONE',  ( 80.00000000000001421, -85.24929059928629727, -32.00000000000000000 ) ) ;
#11513=LINE ( 'NONE', #3369, #8827 ) ;
#11524=ORIENTED_EDGE ( 'NONE', *, *, #2520, .T. ) ;
#11526=CARTESIAN_POINT ( 'NONE',  ( 80.00000000000001421, -85.24929059928629727, -32.00000000000000000 ) ) ;
#11531=EDGE_CURVE ( 'NONE', #81, #1671, #13671, .T. ) ;
#11533=CARTESIAN_POINT ( 'NONE',  ( 80.00000000000001421, -74.24929059928631148, 32.99999999999999289 ) ) ;
#11546=CARTESIAN_POINT ( 'NONE',  ( -80.00000000000001421, -72.24929059928631148, 32.99999999999999289 ) ) ;
#11548=ORIENTED_EDGE ( 'NONE', *, *, #6285, .T. ) ;
#11571=CIRCLE ( 'NONE', #8866, 2.524999999999999467 ) ;
#11581=ORIENTED_EDGE ( 'NONE', *, *, #8512, .F. ) ;
#11590=ADVANCED_FACE ( 'NONE', ( #1417 ), #14425, .F. ) ;
#11595=ORIENTED_EDGE ( 'NONE', *, *, #15099, .F. ) ;
#11615=EDGE_CURVE ( 'NONE', #14077, #12875, #11888, .T. ) ;
#11630=EDGE_CURVE ( 'NONE', #9272, #8897, #10983, .T. ) ;
#11633=DIRECTION ( 'NONE',  ( -0.000000000000000000, 1.000000000000000000, -0.000000000000000000 ) ) ;
#11652=DIRECTION ( 'NONE',  ( 0.000000000000000000, -1.000000000000000000, 0.000000000000000000 ) ) ;
#11655=DIRECTION ( 'NONE',  ( 0.000000000000000000, 0.000000000000000000, 1.000000000000000000 ) ) ;
#11662=DIRECTION ( 'NONE',  ( 0.000000000000000000, 0.000000000000000000, 1.000000000000000000 ) ) ;
#11666=EDGE_CURVE ( 'NONE', #14080, #531, #13637, .T. ) ;
#11673=CARTESIAN_POINT ( 'NONE',  ( -80.00000000000001421, -76.24929059928631148, -4.000000000000000000 ) ) ;
#11698=ORIENTED_EDGE ( 'NONE', *, *, #15129, .F. ) ;
#11701=EDGE_CURVE ( 'NONE', #12443, #3972, #8946, .T. ) ;
#11714=CARTESIAN_POINT ( 'NONE',  ( -65.00000000000001421, -85.27429059928628874, -17.49999999999999645 ) ) ;
#11725=CARTESIAN_POINT ( 'NONE',  ( 65.00000000000001421, -85.24929059928629727, -17.47499999999999787 ) ) ;
#11743=FACE_OUTER_BOUND ( 'NONE', #13460, .T. ) ;
#11754=ORIENTED_EDGE ( 'NONE', *, *, #1843, .F. ) ;
#11763=ORIENTED_EDGE ( 'NONE', *, *, #4031, .T. ) ;
#11777=ORIENTED_EDGE ( 'NONE', *, *, #5459, .F. ) ;
#11796=ORIENTED_EDGE ( 'NONE', *, *, #5463, .T. ) ;
#11809=CARTESIAN_POINT ( 'NONE',  ( 80.00000000000001421, -87.24929059928631148, 35.00000000000000000 ) ) ;
#11820=DIRECTION ( 'NONE',  ( 0.000000000000000000, -1.000000000000000000, 0.000000000000000000 ) ) ;
#11824=PRODUCT_DEFINITION ( 'UNKNOWN', '', #189, #7047 ) ;
#11831=ORIENTED_EDGE ( 'NONE', *, *, #4556, .F. ) ;
#11870=CARTESIAN_POINT ( 'NONE',  ( 80.00000000000001421, -87.24929059928631148, -35.00000000000000000 ) ) ;
#11885=DIRECTION ( 'NONE',  ( 0.000000000000000000, -1.000000000000000000, -1.927470528863119788E-16 ) ) ;
#11888=LINE ( 'NONE', #14205, #10746 ) ;
#11907=EDGE_CURVE ( 'NONE', #14822, #12443, #1090, .T. ) ;
#11933=VERTEX_POINT ( 'NONE', #12013 ) ;
#11938=VECTOR ( 'NONE', #13256, 1000.000000000000000 ) ;
#11943=EDGE_CURVE ( 'NONE', #14405, #1184, #25, .T. ) ;
#11952=EDGE_CURVE ( 'NONE', #8699, #15028, #3639, .T. ) ;
#11973=PLANE ( 'NONE',  #9910 ) ;
#11994=CARTESIAN_POINT ( 'NONE',  ( 80.00000000000001421, -85.24929059928629727, -8.000000000000001776 ) ) ;
#11996=EDGE_CURVE ( 'NONE', #2589, #9131, #4714, .T. ) ;
#12001=DIRECTION ( 'NONE',  ( -0.000000000000000000, 1.000000000000000000, 1.445602896647339163E-16 ) ) ;
#12003=ORIENTED_EDGE ( 'NONE', *, *, #11014, .F. ) ;
#12012=EDGE_CURVE ( 'NONE', #6626, #3181, #9490, .T. ) ;
#12013=CARTESIAN_POINT ( 'NONE',  ( -65.00000000000001421, -87.24929059928631148, -17.50000000000000000 ) ) ;
#12025=CARTESIAN_POINT ( 'NONE',  ( -80.00000000000001421, -74.24929059928631148, -4.000000000000000000 ) ) ;
#12030=PLANE ( 'NONE',  #7668 ) ;
#12034=EDGE_CURVE ( 'NONE', #9345, #7966, #13031, .T. ) ;
#12056=EDGE_CURVE ( 'NONE', #6921, #3262, #5165, .T. ) ;
#12072=EDGE_LOOP ( 'NONE', ( #11524, #12837, #1323, #13377 ) ) ;
#12079=AXIS2_PLACEMENT_3D ( 'NONE', #938, #4487, #5890 ) ;
#12084=ORIENTED_EDGE ( 'NONE', *, *, #395, .T. ) ;
#12087=VECTOR ( 'NONE', #3718, 1000.000000000000000 ) ;
#12100=FACE_OUTER_BOUND ( 'NONE', #4911, .T. ) ;
#12143=ORIENTED_EDGE ( 'NONE', *, *, #12758, .T. ) ;
#12145=FACE_OUTER_BOUND ( 'NONE', #14466, .T. ) ;
#12175=ORIENTED_EDGE ( 'NONE', *, *, #3730, .T. ) ;
#12188=ORIENTED_EDGE ( 'NONE', *, *, #11010, .T. ) ;
#12198=EDGE_LOOP ( 'NONE', ( #6999, #8971, #7896, #6879 ) ) ;
#12202=PLANE ( 'NONE',  #4355 ) ;
#12204=VERTEX_POINT ( 'NONE', #1917 ) ;
#12208=EDGE_LOOP ( 'NONE', ( #6382, #4510 ) ) ;
#12220=DIRECTION ( 'NONE',  ( -0.000000000000000000, -0.000000000000000000, 1.000000000000000000 ) ) ;
#12224=CARTESIAN_POINT ( 'NONE',  ( -80.00000000000001421, -76.24929059928631148, 6.000000000000000000 ) ) ;
#12228=ORIENTED_EDGE ( 'NONE', *, *, #3730, .F. ) ;
#12269=LINE ( 'NONE', #1724, #4735 ) ;
#12286=ORIENTED_EDGE ( 'NONE', *, *, #6273, .T. ) ;
#12287=FACE_OUTER_BOUND ( 'NONE', #13435, .T. ) ;
#12309=CARTESIAN_POINT ( 'NONE',  ( 80.00000000000001421, -85.24929059928629727, -8.000000000000001776 ) ) ;
#12338=VECTOR ( 'NONE', #3692, 1000.000000000000000 ) ;
#12348=LINE ( 'NONE', #7504, #15046 ) ;
#12349=CIRCLE ( 'NONE', #7683, 2.499999999999995115 ) ;
#12361=CARTESIAN_POINT ( 'NONE',  ( 80.00000000000001421, -72.24929059928631148, -32.99999999999999289 ) ) ;
#12362=VECTOR ( 'NONE', #10073, 1000.000000000000000 ) ;
#12363=ORIENTED_EDGE ( 'NONE', *, *, #12731, .T. ) ;
#12366=VERTEX_POINT ( 'NONE', #4618 ) ;
#12378=DIRECTION ( 'NONE',  ( 8.659560562354330119E-17, 0.7071067811865966446, -0.7071067811864982788 ) ) ;
#12384=ORIENTED_EDGE ( 'NONE', *, *, #13851, .T. ) ;
#12418=EDGE_CURVE ( 'NONE', #2170, #14421, #5865, .T. ) ;
#12424=EDGE_CURVE ( 'NONE', #404, #14080, #87, .T. ) ;
#12426=DIRECTION ( 'NONE',  ( -0.000000000000000000, 1.000000000000000000, 1.445602896647339163E-16 ) ) ;
#12441=EDGE_CURVE ( 'NONE', #14421, #10741, #1827, .T. ) ;
#12443=VERTEX_POINT ( 'NONE', #13241 ) ;
#12446=CARTESIAN_POINT ( 'NONE',  ( 80.00000000000001421, -72.24929059928631148, 32.99999999999999289 ) ) ;
#12448=DIRECTION ( 'NONE',  ( 0.000000000000000000, 0.000000000000000000, 1.000000000000000000 ) ) ;
#12471=VECTOR ( 'NONE', #5709, 1000.000000000000000 ) ;
#12474=VERTEX_POINT ( 'NONE', #1750 ) ;
#12497=PLANE ( 'NONE',  #13068 ) ;
#12535=ORIENTED_EDGE ( 'NONE', *, *, #8570, .F. ) ;
#12549=FACE_OUTER_BOUND ( 'NONE', #450, .T. ) ;
#12551=LINE ( 'NONE', #14558, #1046 ) ;
#12555=EDGE_CURVE ( 'NONE', #12474, #11368, #15033, .T. ) ;
#12573=EDGE_CURVE ( 'NONE', #8897, #9272, #10864, .T. ) ;
#12574=ORIENTED_EDGE ( 'NONE', *, *, #15099, .T. ) ;
#12595=EDGE_LOOP ( 'NONE', ( #15132, #227, #9473, #14684 ) ) ;
#12602=VECTOR ( 'NONE', #13044, 1000.000000000000000 ) ;
#12605=DIRECTION ( 'NONE',  ( 0.000000000000000000, 0.000000000000000000, 1.000000000000000000 ) ) ;
#12606=ORIENTED_EDGE ( 'NONE', *, *, #3106, .T. ) ;
#12638=EDGE_LOOP ( 'NONE', ( #10760, #14462 ) ) ;
#12682=CARTESIAN_POINT ( 'NONE',  ( 80.00000000000001421, -87.24929059928631148, -35.00000000000000000 ) ) ;
#12689=VERTEX_POINT ( 'NONE', #3042 ) ;
#12692=DIRECTION ( 'NONE',  ( -0.000000000000000000, 1.000000000000000000, 1.445602896647339163E-16 ) ) ;
#12717=EDGE_CURVE ( 'NONE', #307, #9321, #12348, .T. ) ;
#12731=EDGE_CURVE ( 'NONE', #14173, #4038, #11039, .T. ) ;
#12758=EDGE_CURVE ( 'NONE', #6921, #4603, #12269, .T. ) ;
#12766=CARTESIAN_POINT ( 'NONE',  ( -80.00000000000001421, -74.24929059928631148, -32.00000000000000000 ) ) ;
#12804=DIRECTION ( 'NONE',  ( -0.000000000000000000, 1.000000000000000000, 1.445602896647339163E-16 ) ) ;
#12808=CARTESIAN_POINT ( 'NONE',  ( 80.00000000000001421, -85.24929059928631148, 6.000000000000001776 ) ) ;
#12831=DIRECTION ( 'NONE',  ( 0.000000000000000000, 0.000000000000000000, 1.000000000000000000 ) ) ;
#12837=ORIENTED_EDGE ( 'NONE', *, *, #15073, .F. ) ;
#12841=FACE_OUTER_BOUND ( 'NONE', #1888, .T. ) ;
#12860=VERTEX_POINT ( 'NONE', #6644 ) ;
#12868=EDGE_CURVE ( 'NONE', #7803, #777, #2268, .T. ) ;
#12875=VERTEX_POINT ( 'NONE', #7884 ) ;
#12884=DIRECTION ( 'NONE',  ( -0.000000000000000000, 1.000000000000000000, 1.445602896647339163E-16 ) ) ;
#12896=CARTESIAN_POINT ( 'NONE',  ( -65.00000000000001421, -85.24929059928631148, 19.99999999999999645 ) ) ;
#12897=ORIENTED_EDGE ( 'NONE', *, *, #570, .T. ) ;
#12899=CARTESIAN_POINT ( 'NONE',  ( -80.00000000000001421, -76.24929059928631148, -4.000000000000000000 ) ) ;
#12903=FACE_OUTER_BOUND ( 'NONE', #5232, .T. ) ;
#12914=ORIENTED_EDGE ( 'NONE', *, *, #9328, .F. ) ;
#12941=DIRECTION ( 'NONE',  ( 0.000000000000000000, 1.927470528863120035E-16, -1.000000000000000000 ) ) ;
#12950=CARTESIAN_POINT ( 'NONE',  ( 80.00000000000001421, -74.24929059928631148, 8.000000000000001776 ) ) ;
#12955=DIRECTION ( 'NONE',  ( -1.000000000000000000, -0.000000000000000000, -0.000000000000000000 ) ) ;
#12966=APPLICATION_CONTEXT ( 'automotive_design' ) ;
#13002=EDGE_CURVE ( 'NONE', #5593, #1184, #13119, .T. ) ;
#13009=VERTEX_POINT ( 'NONE', #11725 ) ;
#13031=LINE ( 'NONE', #13107, #866 ) ;
#13037=AXIS2_PLACEMENT_3D ( 'NONE', #12896, #2419, #36 ) ;
#13042=CARTESIAN_POINT ( 'NONE',  ( -80.00000000000001421, -85.24929059928629727, -8.000000000000001776 ) ) ;
#13044=DIRECTION ( 'NONE',  ( 0.000000000000000000, -1.000000000000000000, 0.000000000000000000 ) ) ;
#13050=EDGE_CURVE ( 'NONE', #11368, #12474, #14791, .T. ) ;
#13068=AXIS2_PLACEMENT_3D ( 'NONE', #11183, #4328, #634 ) ;
#13073=ORIENTED_EDGE ( 'NONE', *, *, #13002, .T. ) ;
#13080=AXIS2_PLACEMENT_3D ( 'NONE', #4787, #2164, #5878 ) ;
#13090=PLANE ( 'NONE',  #1452 ) ;
#13101=VECTOR ( 'NONE', #5529, 1000.000000000000000 ) ;
#13107=CARTESIAN_POINT ( 'NONE',  ( -80.00000000000001421, -72.24929059928631148, 34.99999999999999289 ) ) ;
#13118=( NAMED_UNIT ( * ) PLANE_ANGLE_UNIT ( ) SI_UNIT ( $, .RADIAN. ) );
#13119=LINE ( 'NONE', #12899, #2525 ) ;
#13124=AXIS2_PLACEMENT_3D ( 'NONE', #14397, #10857, #10627 ) ;
#13134=ORIENTED_EDGE ( 'NONE', *, *, #14568, .T. ) ;
#13143=EDGE_CURVE ( 'NONE', #15028, #14077, #13329, .T. ) ;
#13176=VECTOR ( 'NONE', #8415, 1000.000000000000000 ) ;
#13188=CARTESIAN_POINT ( 'NONE',  ( 80.00000000000001421, -72.24929059928631148, -34.99999999999999289 ) ) ;
#13200=DIRECTION ( 'NONE',  ( 0.000000000000000000, 0.000000000000000000, 1.000000000000000000 ) ) ;
#13206=FACE_BOUND ( 'NONE', #12638, .T. ) ;
#13213=ORIENTED_EDGE ( 'NONE', *, *, #14361, .T. ) ;
#13214=FACE_OUTER_BOUND ( 'NONE', #15175, .T. ) ;
#13230=ORIENTED_EDGE ( 'NONE', *, *, #13700, .T. ) ;
#13237=CARTESIAN_POINT ( 'NONE',  ( 65.00000000000001421, -87.24929059928631148, -22.49999999999999289 ) ) ;
#13241=CARTESIAN_POINT ( 'NONE',  ( -80.00000000000001421, -74.24929059928631148, 32.00000000000000000 ) ) ;
#13251=VERTEX_POINT ( 'NONE', #14304 ) ;
#13256=DIRECTION ( 'NONE',  ( 0.000000000000000000, 0.000000000000000000, 1.000000000000000000 ) ) ;
#13271=DIRECTION ( 'NONE',  ( 0.000000000000000000, -1.000000000000000000, 0.000000000000000000 ) ) ;
#13276=CARTESIAN_POINT ( 'NONE',  ( 80.00000000000001421, -76.24929059928631148, -4.000000000000000000 ) ) ;
#13284=EDGE_CURVE ( 'NONE', #3110, #2589, #7674, .T. ) ;
#13286=CARTESIAN_POINT ( 'NONE',  ( 80.00000000000001421, -74.24929059928631148, 32.00000000000000000 ) ) ;
#13288=DIRECTION ( 'NONE',  ( 0.000000000000000000, 1.734723475976817547E-15, -1.000000000000000000 ) ) ;
#13289=ORIENTED_EDGE ( 'NONE', *, *, #3385, .T. ) ;
#13311=CARTESIAN_POINT ( 'NONE',  ( -65.00000000000001421, -85.24929059928631148, 22.49999999999999289 ) ) ;
#13315=VECTOR ( 'NONE', #10821, 1000.000000000000000 ) ;
#13317=VECTOR ( 'NONE', #9779, 1000.000000000000000 ) ;
#13318=DIRECTION ( 'NONE',  ( 0.000000000000000000, 0.000000000000000000, 1.000000000000000000 ) ) ;
#13326=DIRECTION ( 'NONE',  ( 0.000000000000000000, -0.000000000000000000, -1.000000000000000000 ) ) ;
#13329=CIRCLE ( 'NONE', #8651, 2.500000000000002220 ) ;
#13335=ORIENTED_EDGE ( 'NONE', *, *, #12418, .F. ) ;
#13346=ORIENTED_EDGE ( 'NONE', *, *, #10701, .F. ) ;
#13377=ORIENTED_EDGE ( 'NONE', *, *, #9328, .T. ) ;
#13395=ADVANCED_FACE ( 'NONE', ( #12145 ), #2679, .F. ) ;
#13403=DIRECTION ( 'NONE',  ( -0.000000000000000000, -0.000000000000000000, -1.000000000000000000 ) ) ;
#13405=DIRECTION ( 'NONE',  ( -0.000000000000000000, -1.000000000000000000, -0.000000000000000000 ) ) ;
#13414=CARTESIAN_POINT ( 'NONE',  ( -80.00000000000001421, -76.24929059928631148, -6.000000000000000000 ) ) ;
#13421=DIRECTION ( 'NONE',  ( 0.000000000000000000, -1.000000000000000000, -1.734723475976817547E-15 ) ) ;
#13432=EDGE_CURVE ( 'NONE', #777, #7803, #11571, .T. ) ;
#13435=EDGE_LOOP ( 'NONE', ( #9627, #2675, #8219, #3589 ) ) ;
#13440=ORIENTED_EDGE ( 'NONE', *, *, #12573, .T. ) ;
#13453=CARTESIAN_POINT ( 'NONE',  ( 80.00000000000001421, -76.24929059928631148, 4.000000000000000000 ) ) ;
#13454=VECTOR ( 'NONE', #5060, 1000.000000000000000 ) ;
#13456=DIRECTION ( 'NONE',  ( 0.000000000000000000, 0.000000000000000000, 1.000000000000000000 ) ) ;
#13457=ORIENTED_EDGE ( 'NONE', *, *, #11378, .F. ) ;
#13460=EDGE_LOOP ( 'NONE', ( #3683, #14853, #13457, #13967 ) ) ;
#13482=LINE ( 'NONE', #7641, #6333 ) ;
#13516=ORIENTED_EDGE ( 'NONE', *, *, #13558, .F. ) ;
#13517=DIRECTION ( 'NONE',  ( 0.000000000000000000, 0.000000000000000000, 1.000000000000000000 ) ) ;
#13538=DIRECTION ( 'NONE',  ( 0.000000000000000000, 0.000000000000000000, 1.000000000000000000 ) ) ;
#13554=LINE ( 'NONE', #14490, #6869 ) ;
#13555=ORIENTED_EDGE ( 'NONE', *, *, #15142, .T. ) ;
#13558=EDGE_CURVE ( 'NONE', #7966, #6896, #5991, .T. ) ;
#13564=AXIS2_PLACEMENT_3D ( 'NONE', #11469, #5727, #2246 ) ;
#13637=LINE ( 'NONE', #7494, #4334 ) ;
#13668=DIRECTION ( 'NONE',  ( 1.000000000000000000, 0.000000000000000000, -0.000000000000000000 ) ) ;
#13671=LINE ( 'NONE', #1966, #5581 ) ;
#13672=LINE ( 'NONE', #11508, #11386 ) ;
#13677=VECTOR ( 'NONE', #592, 1000.000000000000000 ) ;
#13679=LINE ( 'NONE', #5532, #7607 ) ;
#13692=CARTESIAN_POINT ( 'NONE',  ( -65.00000000000001421, -85.24929059928629727, -17.50000000000000000 ) ) ;
#13700=EDGE_CURVE ( 'NONE', #4038, #1083, #9750, .T. ) ;
#13702=VECTOR ( 'NONE', #3514, 1000.000000000000000 ) ;
#13704=DIRECTION ( 'NONE',  ( -0.000000000000000000, 1.000000000000000000, 1.445602896647339163E-16 ) ) ;
#13724=ORIENTED_EDGE ( 'NONE', *, *, #5564, .F. ) ;
#13736=CARTESIAN_POINT ( 'NONE',  ( -80.00000000000001421, -74.24929059928631148, -8.000000000000001776 ) ) ;
#13745=ORIENTED_EDGE ( 'NONE', *, *, #1604, .T. ) ;
#13754=DIRECTION ( 'NONE',  ( 0.000000000000000000, 1.000000000000000000, 0.000000000000000000 ) ) ;
#13769=CARTESIAN_POINT ( 'NONE',  ( 65.00000000000001421, -85.24929059928629727, -19.99999999999999645 ) ) ;
#13779=ORIENTED_EDGE ( 'NONE', *, *, #5040, .F. ) ;
#13799=EDGE_CURVE ( 'NONE', #1184, #4603, #6136, .T. ) ;
#13801=ORIENTED_EDGE ( 'NONE', *, *, #2601, .T. ) ;
#13802=FACE_BOUND ( 'NONE', #1689, .T. ) ;
#13810=DIRECTION ( 'NONE',  ( 0.000000000000000000, 0.000000000000000000, 1.000000000000000000 ) ) ;
#13813=CARTESIAN_POINT ( 'NONE',  ( -80.00000000000001421, -74.24929059928631148, -4.000000000000000000 ) ) ;
#13814=VECTOR ( 'NONE', #8959, 1000.000000000000000 ) ;
#13818=ORIENTED_EDGE ( 'NONE', *, *, #14946, .F. ) ;
#13821=ORIENTED_EDGE ( 'NONE', *, *, #13825, .F. ) ;
#13825=EDGE_CURVE ( 'NONE', #13251, #14077, #280, .T. ) ;
#13829=LINE ( 'NONE', #14900, #14831 ) ;
#13834=AXIS2_PLACEMENT_3D ( 'NONE', #5132, #7512, #9836 ) ;
#13847=AXIS2_PLACEMENT_3D ( 'NONE', #1814, #5281, #2892 ) ;
#13849=FACE_OUTER_BOUND ( 'NONE', #10656, .T. ) ;
#13851=EDGE_CURVE ( 'NONE', #2753, #3756, #5123, .T. ) ;
#13870=ADVANCED_FACE ( 'NONE', ( #14876, #13883, #15040, #13802, #5343 ), #12497, .F. ) ;
#13883=FACE_BOUND ( 'NONE', #1186, .T. ) ;
#13912=CARTESIAN_POINT ( 'NONE',  ( -80.00000000000001421, -85.24929059928631148, -6.000000000000001776 ) ) ;
#13914=ORIENTED_EDGE ( 'NONE', *, *, #1479, .F. ) ;
#13919=ORIENTED_EDGE ( 'NONE', *, *, #6790, .T. ) ;
#13921=LINE ( 'NONE', #4379, #14176 ) ;
#13931=CARTESIAN_POINT ( 'NONE',  ( 80.00000000000001421, -72.24929059928631148, 34.99999999999999289 ) ) ;
#13943=CARTESIAN_POINT ( 'NONE',  ( -65.00000000000001421, -85.24929059928629727, -17.47499999999999787 ) ) ;
#13957=CARTESIAN_POINT ( 'NONE',  ( -65.00000000000001421, -85.27429059928630295, 17.49999999999999645 ) ) ;
#13959=CIRCLE ( 'NONE', #9029, 2.499999999999995115 ) ;
#13960=ORIENTED_EDGE ( 'NONE', *, *, #11014, .T. ) ;
#13967=ORIENTED_EDGE ( 'NONE', *, *, #5512, .T. ) ;
#13982=CARTESIAN_POINT ( 'NONE',  ( -80.00000000000001421, -87.24929059928631148, 35.00000000000000000 ) ) ;
#13993=PLANE ( 'NONE',  #10754 ) ;
#13997=ORIENTED_EDGE ( 'NONE', *, *, #1430, .F. ) ;
#14000=DIRECTION ( 'NONE',  ( 0.000000000000000000, 0.000000000000000000, 1.000000000000000000 ) ) ;
#14001=ORIENTED_EDGE ( 'NONE', *, *, #13002, .F. ) ;
#14006=ORIENTED_EDGE ( 'NONE', *, *, #5658, .T. ) ;
#14023=CARTESIAN_POINT ( 'NONE',  ( 80.00000000000001421, -72.24929059928631148, 34.99999999999999289 ) ) ;
#14043=CARTESIAN_POINT ( 'NONE',  ( 80.00000000000001421, -76.24929059928631148, 6.000000000000000000 ) ) ;
#14058=EDGE_LOOP ( 'NONE', ( #5777, #14647 ) ) ;
#14077=VERTEX_POINT ( 'NONE', #2186 ) ;
#14080=VERTEX_POINT ( 'NONE', #13042 ) ;
#14086=ORIENTED_EDGE ( 'NONE', *, *, #13851, .F. ) ;
#14089=CARTESIAN_POINT ( 'NONE',  ( -65.00000000000001421, -85.24929059928631148, 22.52499999999999503 ) ) ;
#14097=AXIS2_PLACEMENT_3D ( 'NONE', #14836, #11149, #12448 ) ;
#14115=EDGE_LOOP ( 'NONE', ( #6508, #9413, #12535, #7885 ) ) ;
#14123=LINE ( 'NONE', #1413, #4491 ) ;
#14126=DIRECTION ( 'NONE',  ( -1.000000000000000000, -0.000000000000000000, -0.000000000000000000 ) ) ;
#14140=EDGE_CURVE ( 'NONE', #1580, #5593, #14422, .T. ) ;
#14145=CARTESIAN_POINT ( 'NONE',  ( 80.00000000000001421, -87.24929059928631148, 35.00000000000000000 ) ) ;
#14148=CARTESIAN_POINT ( 'NONE',  ( 80.00000000000001421, -74.24929059928631148, -32.99999999999999289 ) ) ;
#14166=VECTOR ( 'NONE', #8023, 1000.000000000000000 ) ;
#14171=MANIFOLD_SOLID_BREP ( 'Body-Move/Copy1', #5298 ) ;
#14173=VERTEX_POINT ( 'NONE', #13188 ) ;
#14176=VECTOR ( 'NONE', #14845, 1000.000000000000000 ) ;
#14178=EDGE_CURVE ( 'NONE', #9131, #1671, #14492, .T. ) ;
#14183=DIRECTION ( 'NONE',  ( 0.000000000000000000, -0.000000000000000000, -1.000000000000000000 ) ) ;
#14203=AXIS2_PLACEMENT_3D ( 'NONE', #9398, #12941, #2151 ) ;
#14205=CARTESIAN_POINT ( 'NONE',  ( 65.00000000000001421, -85.24929059928631148, 22.52499999999999503 ) ) ;
#14207=CARTESIAN_POINT ( 'NONE',  ( -80.00000000000001421, -87.24929059928631148, -35.00000000000000000 ) ) ;
#14224=EDGE_CURVE ( 'NONE', #13251, #8699, #6682, .T. ) ;
#14225=DIRECTION ( 'NONE',  ( 0.000000000000000000, 0.000000000000000000, 1.000000000000000000 ) ) ;
#14226=CARTESIAN_POINT ( 'NONE',  ( -65.00000000000001421, -85.27429059928628874, -22.50000000000000000 ) ) ;
#14253=DIRECTION ( 'NONE',  ( -0.000000000000000000, 1.000000000000000000, 1.445602896647339163E-16 ) ) ;
#14275=CARTESIAN_POINT ( 'NONE',  ( 80.00000000000001421, -76.24929059928631148, -4.000000000000000000 ) ) ;
#14282=ORIENTED_EDGE ( 'NONE', *, *, #11952, .T. ) ;
#14304=CARTESIAN_POINT ( 'NONE',  ( 65.00000000000001421, -87.24929059928631148, 22.49999999999999289 ) ) ;
#14307=VERTEX_POINT ( 'NONE', #12950 ) ;
#14331=FACE_OUTER_BOUND ( 'NONE', #10997, .T. ) ;
#14342=ADVANCED_FACE ( 'NONE', ( #1316 ), #8335, .F. ) ;
#14346=VECTOR ( 'NONE', #6093, 1000.000000000000000 ) ;
#14357=VECTOR ( 'NONE', #9303, 1000.000000000000000 ) ;
#14361=EDGE_CURVE ( 'NONE', #3181, #3011, #15103, .T. ) ;
#14363=DIRECTION ( 'NONE',  ( 0.000000000000000000, 1.000000000000000000, 0.000000000000000000 ) ) ;
#14380=ORIENTED_EDGE ( 'NONE', *, *, #13143, .T. ) ;
#14383=ORIENTED_EDGE ( 'NONE', *, *, #11036, .F. ) ;
#14397=CARTESIAN_POINT ( 'NONE',  ( -65.00000000000001421, -85.24929059928629727, -19.99999999999999645 ) ) ;
#14405=VERTEX_POINT ( 'NONE', #3996 ) ;
#14411=PLANE ( 'NONE',  #9808 ) ;
#14421=VERTEX_POINT ( 'NONE', #4936 ) ;
#14422=LINE ( 'NONE', #12025, #12087 ) ;
#14425=PLANE ( 'NONE',  #1644 ) ;
#14426=CARTESIAN_POINT ( 'NONE',  ( 80.00000000000001421, -74.24929059928631148, -8.000000000000001776 ) ) ;
#14433=ORIENTED_EDGE ( 'NONE', *, *, #4577, .T. ) ;
#14447=ORIENTED_EDGE ( 'NONE', *, *, #6244, .F. ) ;
#14460=ORIENTED_EDGE ( 'NONE', *, *, #14866, .T. ) ;
#14462=ORIENTED_EDGE ( 'NONE', *, *, #6884, .F. ) ;
#14466=EDGE_LOOP ( 'NONE', ( #7685, #10848, #1683, #13801 ) ) ;
#14471=CARTESIAN_POINT ( 'NONE',  ( -65.00000000000001421, -85.24929059928629727, -22.49999999999999289 ) ) ;
#14473=ADVANCED_FACE ( 'NONE', ( #14331 ), #9644, .T. ) ;
#14481=CARTESIAN_POINT ( 'NONE',  ( -65.00000000000001421, -87.24929059928631148, 19.99999999999999645 ) ) ;
#14490=CARTESIAN_POINT ( 'NONE',  ( -80.00000000000001421, -74.24929059928631148, -32.00000000000000000 ) ) ;
#14492=LINE ( 'NONE', #7559, #1999 ) ;
#14506=DIRECTION ( 'NONE',  ( -0.000000000000000000, 1.000000000000000000, -0.000000000000000000 ) ) ;
#14517=DIRECTION ( 'NONE',  ( 0.000000000000000000, 0.000000000000000000, 1.000000000000000000 ) ) ;
#14518=ORIENTED_EDGE ( 'NONE', *, *, #14178, .T. ) ;
#14522=ORIENTED_EDGE ( 'NONE', *, *, #11531, .F. ) ;
#14524=ORIENTED_EDGE ( 'NONE', *, *, #2357, .T. ) ;
#14534=EDGE_CURVE ( 'NONE', #2944, #5593, #2700, .T. ) ;
#14537=DIRECTION ( 'NONE',  ( -0.000000000000000000, -0.000000000000000000, 1.000000000000000000 ) ) ;
#14552=ORIENTED_EDGE ( 'NONE', *, *, #5136, .T. ) ;
#14558=CARTESIAN_POINT ( 'NONE',  ( 65.00000000000001421, -85.24929059928629727, -22.49999999999999289 ) ) ;
#14568=EDGE_CURVE ( 'NONE', #7720, #246, #5385, .T. ) ;
#14591=EDGE_CURVE ( 'NONE', #11933, #3181, #8922, .T. ) ;
#14599=DIRECTION ( 'NONE',  ( -0.000000000000000000, 1.445602896647339163E-16, 1.000000000000000000 ) ) ;
#14621=DIRECTION ( 'NONE',  ( 0.000000000000000000, 0.000000000000000000, 1.000000000000000000 ) ) ;
#14647=ORIENTED_EDGE ( 'NONE', *, *, #737, .F. ) ;
#14659=LINE ( 'NONE', #6581, #13454 ) ;
#14665=DIRECTION ( 'NONE',  ( -1.000000000000000000, -0.000000000000000000, -0.000000000000000000 ) ) ;
#14667=DIRECTION ( 'NONE',  ( -0.000000000000000000, 1.000000000000000000, 1.445602896647339163E-16 ) ) ;
#14678=CARTESIAN_POINT ( 'NONE',  ( 80.00000000000001421, -74.24929059928631148, 8.000000000000001776 ) ) ;
#14684=ORIENTED_EDGE ( 'NONE', *, *, #7910, .T. ) ;
#14697=ORIENTED_EDGE ( 'NONE', *, *, #10557, .T. ) ;
#14735=CARTESIAN_POINT ( 'NONE',  ( 80.00000000000001421, -87.24929059928629727, 0.000000000000000000 ) ) ;
#14739=CARTESIAN_POINT ( 'NONE',  ( 65.00000000000001421, -85.27429059928630295, 19.99999999999999645 ) ) ;
#14741=ORIENTED_EDGE ( 'NONE', *, *, #11378, .T. ) ;
#14758=EDGE_CURVE ( 'NONE', #1978, #5126, #9901, .T. ) ;
#14766=LINE ( 'NONE', #11526, #14937 ) ;
#14791=CIRCLE ( 'NONE', #3734, 2.499999999999995115 ) ;
#14804=CARTESIAN_POINT ( 'NONE',  ( 65.00000000000001421, -85.24929059928629727, -17.50000000000000000 ) ) ;
#14805=CARTESIAN_POINT ( 'NONE',  ( 80.00000000000001421, -85.24929059928629727, -32.00000000000000000 ) ) ;
#14806=EDGE_CURVE ( 'NONE', #14173, #14421, #10044, .T. ) ;
#14822=VERTEX_POINT ( 'NONE', #13286 ) ;
#14829=DIRECTION ( 'NONE',  ( -0.000000000000000000, 1.000000000000000000, -0.000000000000000000 ) ) ;
#14831=VECTOR ( 'NONE', #1825, 1000.000000000000000 ) ;
#14836=CARTESIAN_POINT ( 'NONE',  ( -65.00000000000001421, -85.24929059928631148, 19.99999999999999645 ) ) ;
#14842=ORIENTED_EDGE ( 'NONE', *, *, #1843, .T. ) ;
#14845=DIRECTION ( 'NONE',  ( 0.000000000000000000, -1.734723475976817547E-15, 1.000000000000000000 ) ) ;
#14853=ORIENTED_EDGE ( 'NONE', *, *, #3435, .F. ) ;
#14866=EDGE_CURVE ( 'NONE', #12474, #4665, #11490, .T. ) ;
#14876=FACE_BOUND ( 'NONE', #11489, .T. ) ;
#14880=FACE_OUTER_BOUND ( 'NONE', #14913, .T. ) ;
#14895=ORIENTED_EDGE ( 'NONE', *, *, #6244, .T. ) ;
#14900=CARTESIAN_POINT ( 'NONE',  ( 80.00000000000001421, -85.24929059928629727, 8.000000000000001776 ) ) ;
#14913=EDGE_LOOP ( 'NONE', ( #14433, #3956, #1274, #2158 ) ) ;
#14926=ORIENTED_EDGE ( 'NONE', *, *, #4967, .F. ) ;
#14937=VECTOR ( 'NONE', #6840, 1000.000000000000000 ) ;
#14942=DIRECTION ( 'NONE',  ( 0.000000000000000000, 0.000000000000000000, -1.000000000000000000 ) ) ;
#14946=EDGE_CURVE ( 'NONE', #307, #4665, #10887, .T. ) ;
#14950=CONICAL_SURFACE ( 'NONE', #7338, 2.524999999999999467, 0.7853981633973787790 ) ;
#14953=LINE ( 'NONE', #4402, #1706 ) ;
#14994=LINE ( 'NONE', #13912, #14357 ) ;
#15002=LINE ( 'NONE', #8923, #1668 ) ;
#15011=CARTESIAN_POINT ( 'NONE',  ( 80.00000000000001421, -87.24929059928631148, -35.00000000000000000 ) ) ;
#15015=CARTESIAN_POINT ( 'NONE',  ( -65.00000000000001421, -87.24929059928631148, 17.50000000000000000 ) ) ;
#15026=LINE ( 'NONE', #11546, #11488 ) ;
#15028=VERTEX_POINT ( 'NONE', #5816 ) ;
#15033=CIRCLE ( 'NONE', #8883, 2.499999999999995115 ) ;
#15035=CARTESIAN_POINT ( 'NONE',  ( 80.00000000000001421, -72.24929059928631148, -32.99999999999999289 ) ) ;
#15040=FACE_BOUND ( 'NONE', #2547, .T. ) ;
#15042=EDGE_LOOP ( 'NONE', ( #9527, #10687 ) ) ;
#15046=VECTOR ( 'NONE', #712, 1000.000000000000114 ) ;
#15047=VECTOR ( 'NONE', #4619, 1000.000000000000000 ) ;
#15061=EDGE_LOOP ( 'NONE', ( #8092, #11831, #5268, #8259 ) ) ;
#15068=DIRECTION ( 'NONE',  ( -0.000000000000000000, 1.000000000000000000, 0.000000000000000000 ) ) ;
#15073=EDGE_CURVE ( 'NONE', #1083, #11420, #8118, .T. ) ;
#15084=CIRCLE ( 'NONE', #3037, 2.500000000000002220 ) ;
#15099=EDGE_CURVE ( 'NONE', #14405, #6921, #14123, .T. ) ;
#15100=DIRECTION ( 'NONE',  ( -0.000000000000000000, 1.000000000000000000, -0.000000000000000000 ) ) ;
#15103=LINE ( 'NONE', #13943, #11344 ) ;
#15106=ORIENTED_EDGE ( 'NONE', *, *, #12758, .F. ) ;
#15129=EDGE_CURVE ( 'NONE', #12366, #12204, #2344, .T. ) ;
#15132=ORIENTED_EDGE ( 'NONE', *, *, #11952, .F. ) ;
#15142=EDGE_CURVE ( 'NONE', #3601, #9272, #8205, .T. ) ;
#15161=CARTESIAN_POINT ( 'NONE',  ( -80.00000000000001421, -76.24929059928631148, 6.000000000000000000 ) ) ;
#15173=ORIENTED_EDGE ( 'NONE', *, *, #6572, .T. ) ;
#15175=EDGE_LOOP ( 'NONE', ( #15220, #12914, #3822, #6257 ) ) ;
#15178=PLANE ( 'NONE',  #4482 ) ;
#15199=DIRECTION ( 'NONE',  ( -0.000000000000000000, 1.927470528863120035E-16, 1.000000000000000000 ) ) ;
#15212=ORIENTED_EDGE ( 'NONE', *, *, #11377, .T. ) ;
#15220=ORIENTED_EDGE ( 'NONE', *, *, #12441, .T. ) ;
#15221=ORIENTED_EDGE ( 'NONE', *, *, #950, .F. ) ;
#15225=DIRECTION ( 'NONE',  ( -0.000000000000000000, 0.000000000000000000, 1.000000000000000000 ) ) ;
#15226=CIRCLE ( 'NONE', #3676, 2.524999999999999467 ) ;
#15238=COLOUR_RGB('Dark Blue',0.08,0.2,0.34);
#15239=FILL_AREA_STYLE_COLOUR('',#15238);
#15240=FILL_AREA_STYLE('',(#15239));
#15241=SURFACE_STYLE_FILL_AREA(#15240);
#15242=SURFACE_SIDE_STYLE('',(#15241));
#15243=SURFACE_STYLE_USAGE(.BOTH.,#15242);
#15244=PRESENTATION_STYLE_ASSIGNMENT((#15243));
ENDSEC;
END-ISO-10303-21;
